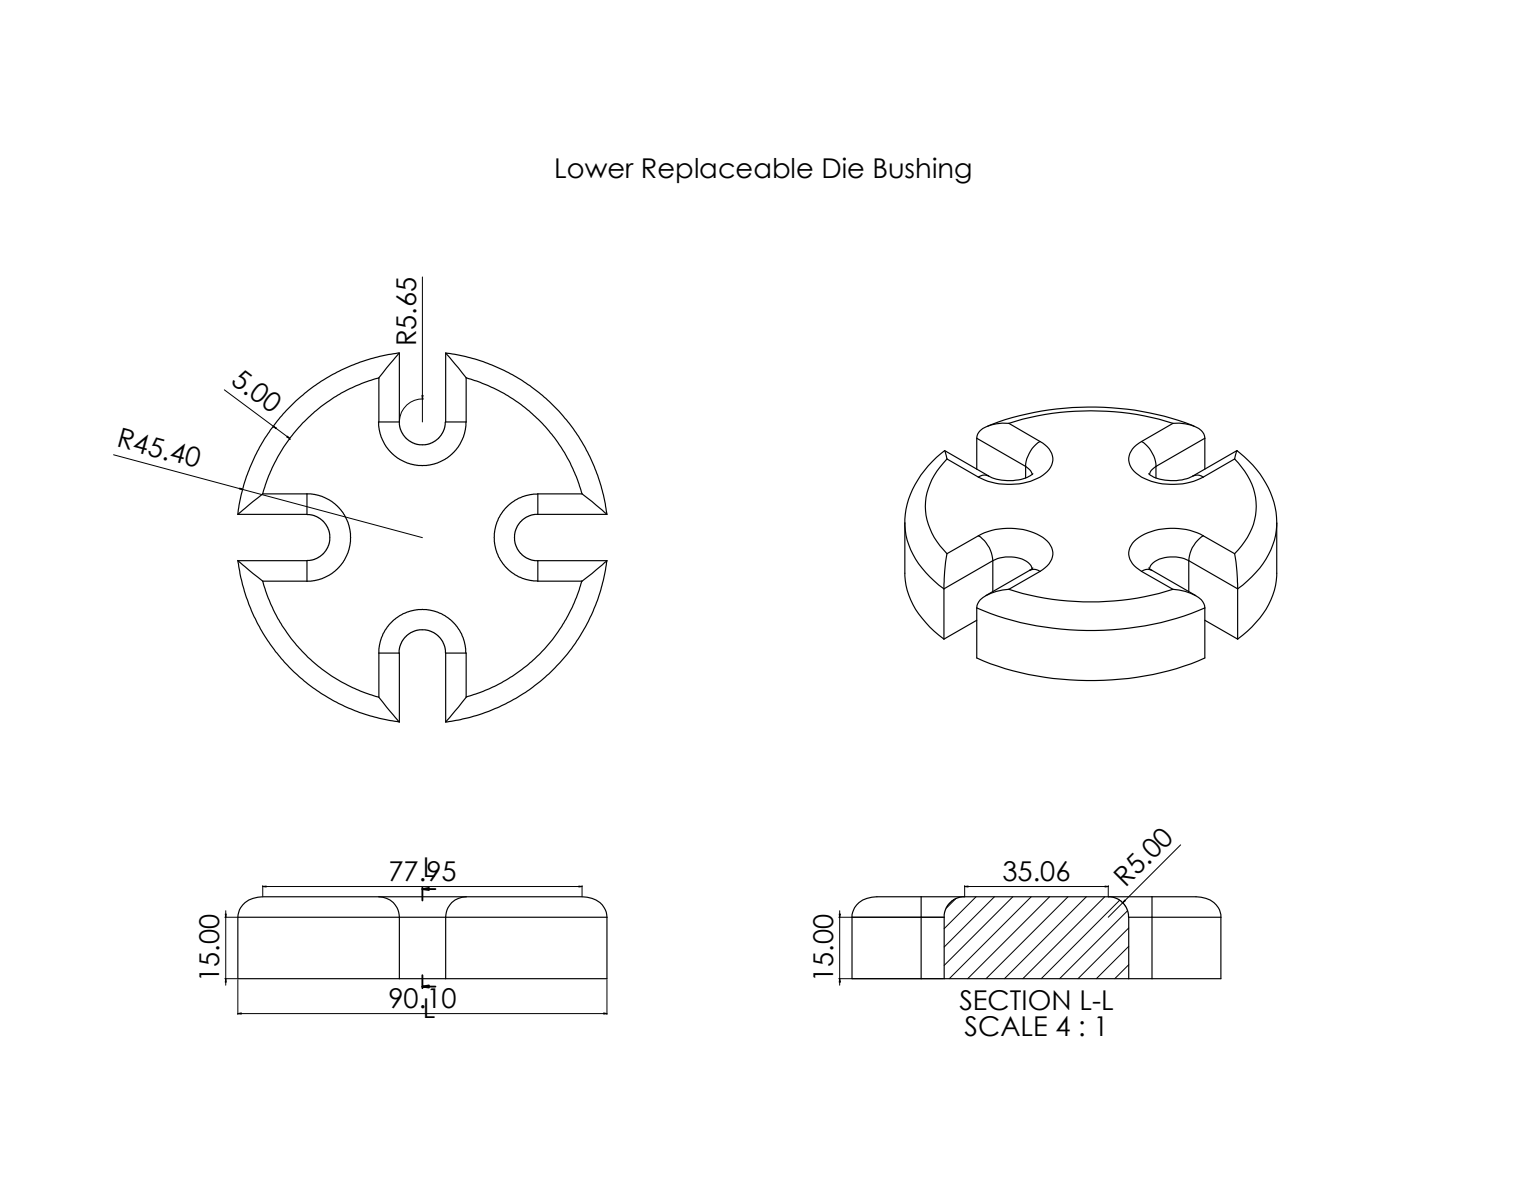
ISO-10303-21;
HEADER;
FILE_DESCRIPTION (('STEP AP214'),
    '1' );
FILE_NAME ('Lower Replaceable Die Bushing.step',
    '2026-10-21T18:33:49',
    ( '' ),
    ( '' ),
    'SwSTEP 2.0',
    'SolidWorks 2025',
    '' );
FILE_SCHEMA (( 'AUTOMOTIVE_DESIGN' ));
ENDSEC;

DATA;
#18=CARTESIAN_POINT ( 'NONE',  ( -78.51801170372752381, -91.96846159163192169, 42.55230335834794175 ) ) ;
#24=CARTESIAN_POINT ( 'NONE',  ( -110.0337185876616815, -91.08930958056578220, -10.39386245929468444 ) ) ;
#38=CARTESIAN_POINT ( 'NONE',  ( -27.30335599338096841, -92.58099833983887095, 7.070576347711331699 ) ) ;
#39=DIRECTION ( 'NONE',  ( 3.469446951953611033E-15, 0.000000000000000000, -1.000000000000000000 ) ) ;
#48=DIRECTION ( 'NONE',  ( -1.000000000000000000, 0.000000000000000000, 0.000000000000000000 ) ) ;
#60=VERTEX_POINT ( 'NONE', #5921 ) ;
#117=DIRECTION ( 'NONE',  ( 0.000000000000000000, 1.000000000000000000, -0.000000000000000000 ) ) ;
#121=CARTESIAN_POINT ( 'NONE',  ( -115.7702289486887537, -95.65021661331556402, -5.654315315326000402 ) ) ;
#129=FACE_OUTER_BOUND ( 'NONE', #15736, .T. ) ;
#153=ORIENTED_EDGE ( 'NONE', *, *, #7643, .F. ) ;
#166=PLANE ( 'NONE',  #9698 ) ;
#184=CARTESIAN_POINT ( 'NONE',  ( -64.80066835027049876, -94.42547236494613117, -44.74948972093426391 ) ) ;
#208=CARTESIAN_POINT ( 'NONE',  ( -80.32997185471272417, -91.18731257919070288, 40.31990080433438095 ) ) ;
#212=CARTESIAN_POINT ( 'NONE',  ( -114.8884567811962967, -93.39009998357855125, -6.425136209964025902 ) ) ;
#215=ADVANCED_FACE ( 'NONE', ( #695 ), #10288, .T. ) ;
#221=CARTESIAN_POINT ( 'NONE',  ( -81.37409655828265898, -96.08423613455721579, -2.623087607583323579E-13 ) ) ;
#233=EDGE_CURVE ( 'NONE', #4074, #17713, #2000, .T. ) ;
#247=EDGE_LOOP ( 'NONE', ( #1699, #2209, #13687, #4336 ) ) ;
#251=AXIS2_PLACEMENT_3D ( 'NONE', #13885, #4066, #1079 ) ;
#273=ORIENTED_EDGE ( 'NONE', *, *, #7918, .F. ) ;
#275=ORIENTED_EDGE ( 'NONE', *, *, #8832, .T. ) ;
#285=CARTESIAN_POINT ( 'NONE',  ( -80.85270481229034090, -91.10977358899566525, 39.65137850708985923 ) ) ;
#290=DIRECTION ( 'NONE',  ( 0.000000000000000000, 1.000000000000000000, -0.000000000000000000 ) ) ;
#336=CARTESIAN_POINT ( 'NONE',  ( 0.000000000000000000, -111.0842361345572158, 0.000000000000000000 ) ) ;
#343=DIRECTION ( 'NONE',  ( -0.000000000000000000, -1.000000000000000000, 0.000000000000000000 ) ) ;
#373=ADVANCED_FACE ( 'NONE', ( #129 ), #745, .T. ) ;
#380=CARTESIAN_POINT ( 'NONE',  ( -81.37409655828265898, -96.08423613455721579, -8.525034724645805924E-13 ) ) ;
#398=LINE ( 'NONE', #4246, #4265 ) ;
#400=CARTESIAN_POINT ( 'NONE',  ( -28.16748190072492974, -91.96845925178433845, 7.798233810088259332 ) ) ;
#432=VECTOR ( 'NONE', #18327, 1000.000000000000000 ) ;
#460=DIRECTION ( 'NONE',  ( -0.000000000000000000, -1.000000000000000000, -0.000000000000000000 ) ) ;
#467=ORIENTED_EDGE ( 'NONE', *, *, #4024, .T. ) ;
#480=CARTESIAN_POINT ( 'NONE',  ( -76.37409655828265898, -111.0842361345572158, -2.461913000519969422E-13 ) ) ;
#513=VERTEX_POINT ( 'NONE', #15067 ) ;
#516=ORIENTED_EDGE ( 'NONE', *, *, #6768, .F. ) ;
#582=DIRECTION ( 'NONE',  ( -1.000000000000000000, 0.000000000000000000, -6.950654929607132427E-15 ) ) ;
#614=ORIENTED_EDGE ( 'NONE', *, *, #15108, .F. ) ;
#620=CYLINDRICAL_SURFACE ( 'NONE', #5187, 5.654315315325682434 ) ;
#640=CARTESIAN_POINT ( 'NONE',  ( -42.53669312409158465, -96.08423613455721579, 5.204170427930421283E-15 ) ) ;
#642=EDGE_CURVE ( 'NONE', #11067, #11836, #18161, .T. ) ;
#660=CARTESIAN_POINT ( 'NONE',  ( -98.90286936182226896, -91.08423613455721579, -10.65431531532588316 ) ) ;
#662=CARTESIAN_POINT ( 'NONE',  ( -76.37409655828280108, -111.0842361345572158, 45.05044770573179846 ) ) ;
#690=ADVANCED_FACE ( 'NONE', ( #9649 ), #1237, .F. ) ;
#695=FACE_OUTER_BOUND ( 'NONE', #12047, .T. ) ;
#696=CARTESIAN_POINT ( 'NONE',  ( -42.53669312409158465, -96.08423613455721579, 5.204170427930421283E-15 ) ) ;
#701=DIRECTION ( 'NONE',  ( -0.000000000000000000, -1.000000000000000000, -0.000000000000000000 ) ) ;
#705=DIRECTION ( 'NONE',  ( 0.000000000000000000, 0.000000000000000000, 1.000000000000000000 ) ) ;
#745=TOROIDAL_SURFACE ( 'NONE', #11214, 40.40389983439752086, 5.000000000000000000 ) ;
#749=VECTOR ( 'NONE', #11083, 1000.000000000000000 ) ;
#759=DIRECTION ( 'NONE',  ( 9.117856171852156377E-15, 0.000000000000000000, 1.000000000000000000 ) ) ;
#763=CARTESIAN_POINT ( 'NONE',  ( -31.57667891805219895, -91.08423613455724421, -10.52509945732311891 ) ) ;
#787=EDGE_LOOP ( 'NONE', ( #8636, #4060, #891, #3393 ) ) ;
#799=DIRECTION ( 'NONE',  ( 1.000000000000000000, 0.000000000000000000, -0.000000000000000000 ) ) ;
#800=VERTEX_POINT ( 'NONE', #13028 ) ;
#830=ORIENTED_EDGE ( 'NONE', *, *, #10988, .T. ) ;
#836=LINE ( 'NONE', #4020, #9670 ) ;
#853=DIRECTION ( 'NONE',  ( 0.000000000000000000, 1.000000000000000000, -0.000000000000000000 ) ) ;
#867=B_SPLINE_CURVE_WITH_KNOTS ( 'NONE', 3,
 ( #14957, #763, #6351, #1047, #10957, #8142, #9362, #2435, #16641, #15059, #7957, #5140, #10857, #13758, #16454, #9455, #18156, #6644, #12083, #12462 ),
 .UNSPECIFIED., .F., .F.,
 ( 4, 2, 2, 2, 2, 2, 2, 2, 2, 4 ),
 ( -1.439925654488394098E-05, 0.0006244272253376518481, 0.001263253707220187783, 0.002540906670985255533, 0.003818559634750323065, 0.005096212598515390164, 0.006373865562280457697, 0.007651518526045524363, 0.008929171489810592763, 0.01020682445357565943 ),
 .UNSPECIFIED. ) ;
#875=CARTESIAN_POINT ( 'NONE',  ( -70.71978124295696944, -96.08423613455721579, 5.204170427930421283E-15 ) ) ;
#888=CARTESIAN_POINT ( 'NONE',  ( -81.11364370225096820, -91.08930958056581062, -39.31393734470488255 ) ) ;
#891=ORIENTED_EDGE ( 'NONE', *, *, #12147, .T. ) ;
#911=VECTOR ( 'NONE', #6055, 1000.000000000000000 ) ;
#939=EDGE_CURVE ( 'NONE', #10198, #60, #13560, .T. ) ;
#966=CARTESIAN_POINT ( 'NONE',  ( -115.7702289486888247, -96.08423613455721579, 5.654315315325360913 ) ) ;
#976=CYLINDRICAL_SURFACE ( 'NONE', #17426, 45.40389983439752086 ) ;
#1015=CARTESIAN_POINT ( 'NONE',  ( -60.06546592763143622, -91.08423613455721579, 38.97384619189705290 ) ) ;
#1016=CARTESIAN_POINT ( 'NONE',  ( -63.40980125876075135, -92.35432432510552303, 43.13417342538335930 ) ) ;
#1043=DIRECTION ( 'NONE',  ( 0.000000000000000000, 1.000000000000000000, -0.000000000000000000 ) ) ;
#1047=CARTESIAN_POINT ( 'NONE',  ( -31.06841040534018106, -91.10977296152353233, -10.13292952605206310 ) ) ;
#1055=ADVANCED_FACE ( 'NONE', ( #3537 ), #14940, .T. ) ;
#1058=UNCERTAINTY_MEASURE_WITH_UNIT (LENGTH_MEASURE( 1.000000000000000082E-05 ), #12203, 'distance_accuracy_value', 'NONE');
#1079=DIRECTION ( 'NONE',  ( 0.000000000000000000, 0.000000000000000000, -1.000000000000000000 ) ) ;
#1087=CARTESIAN_POINT ( 'NONE',  ( -70.71978124295668522, -96.08423613455721579, -17.52877280353970235 ) ) ;
#1089=CARTESIAN_POINT ( 'NONE',  ( -30.06971094502080177, -91.24992749556385263, 9.348345296714491326 ) ) ;
#1115=VERTEX_POINT ( 'NONE', #16826 ) ;
#1116=CARTESIAN_POINT ( 'NONE',  ( -62.67046908522836191, -91.80659809767264790, 42.25010775664332385 ) ) ;
#1128=DIRECTION ( 'NONE',  ( -0.000000000000000000, -1.000000000000000000, -0.000000000000000000 ) ) ;
#1157=CARTESIAN_POINT ( 'NONE',  ( -70.71978124295696944, -96.08423613455721579, 5.204170427930421283E-15 ) ) ;
#1166=DIRECTION ( 'NONE',  ( 0.000000000000000000, 0.000000000000000000, 1.000000000000000000 ) ) ;
#1214=DIRECTION ( 'NONE',  ( 0.000000000000000000, -0.000000000000000000, 1.000000000000000000 ) ) ;
#1237=CYLINDRICAL_SURFACE ( 'NONE', #13579, 5.654315315325682434 ) ;
#1244=ORIENTED_EDGE ( 'NONE', *, *, #8704, .T. ) ;
#1273=LINE ( 'NONE', #6877, #3065 ) ;
#1297=DIRECTION ( 'NONE',  ( 0.000000000000000000, 0.000000000000000000, 1.000000000000000000 ) ) ;
#1307=EDGE_CURVE ( 'NONE', #800, #4074, #8827, .T. ) ;
#1325=LINE ( 'NONE', #9738, #8125 ) ;
#1351=ORIENTED_EDGE ( 'NONE', *, *, #2145, .T. ) ;
#1352=AXIS2_PLACEMENT_3D ( 'NONE', #4171, #12879, #17171 ) ;
#1385=DIRECTION ( 'NONE',  ( -0.000000000000000000, -1.000000000000000000, -0.000000000000000000 ) ) ;
#1398=LINE ( 'NONE', #18508, #12882 ) ;
#1404=ORIENTED_EDGE ( 'NONE', *, *, #16960, .T. ) ;
#1408=CARTESIAN_POINT ( 'NONE',  ( -62.15805688404110185, -91.53392936304808813, -41.62626455281442617 ) ) ;
#1453=LINE ( 'NONE', #7252, #16398 ) ;
#1518=CARTESIAN_POINT ( 'NONE',  ( -98.90286936182226896, -96.08423613455721579, -10.65431531532588494 ) ) ;
#1520=CARTESIAN_POINT ( 'NONE',  ( -80.06812138002696599, -91.24992890033500714, 40.65007677557128574 ) ) ;
#1528=ADVANCED_FACE ( 'NONE', ( #17112 ), #14234, .T. ) ;
#1541=AXIS2_PLACEMENT_3D ( 'NONE', #17995, #9123, #14899 ) ;
#1567=DIRECTION ( 'NONE',  ( 0.000000000000000000, 0.000000000000000000, 1.000000000000000000 ) ) ;
#1571=CARTESIAN_POINT ( 'NONE',  ( -65.06546592763082515, -91.08423613455721579, -45.05044770573174873 ) ) ;
#1577=ORIENTED_EDGE ( 'NONE', *, *, #16595, .T. ) ;
#1615=CARTESIAN_POINT ( 'NONE',  ( -111.0396820472913220, -91.18731257919070288, -9.610190611755886181 ) ) ;
#1629=EDGE_LOOP ( 'NONE', ( #8679, #16373, #14384, #17205 ) ) ;
#1647=CARTESIAN_POINT ( 'NONE',  ( -76.37409655828275845, -96.08423613455721579, 28.18308811886536347 ) ) ;
#1699=ORIENTED_EDGE ( 'NONE', *, *, #16467, .T. ) ;
#1712=DIRECTION ( 'NONE',  ( 0.000000000000000000, 0.000000000000000000, 1.000000000000000000 ) ) ;
#1713=FACE_OUTER_BOUND ( 'NONE', #7475, .T. ) ;
#1732=DIRECTION ( 'NONE',  ( -1.000000000000000000, 0.000000000000000000, -3.223492141267075737E-15 ) ) ;
#1740=PLANE ( 'NONE',  #13721 ) ;
#1746=DIRECTION ( 'NONE',  ( -0.000000000000000000, -1.000000000000000000, -0.000000000000000000 ) ) ;
#1774=CYLINDRICAL_SURFACE ( 'NONE', #16267, 4.999999999999997335 ) ;
#1778=ADVANCED_FACE ( 'NONE', ( #3809 ), #13608, .T. ) ;
#1780=CARTESIAN_POINT ( 'NONE',  ( -79.54423376290981196, -91.42293805878658475, 41.30286037549874578 ) ) ;
#1781=VECTOR ( 'NONE', #15202, 1000.000000000000000 ) ;
#1822=ORIENTED_EDGE ( 'NONE', *, *, #10528, .T. ) ;
#1840=DIRECTION ( 'NONE',  ( 0.000000000000000000, 0.000000000000000000, 1.000000000000000000 ) ) ;
#1855=ADVANCED_FACE ( 'NONE', ( #17513 ), #8919, .T. ) ;
#1891=DIRECTION ( 'NONE',  ( 0.000000000000000000, 0.000000000000000000, 1.000000000000000000 ) ) ;
#1942=EDGE_CURVE ( 'NONE', #14058, #17058, #10586, .T. ) ;
#1992=CARTESIAN_POINT ( 'NONE',  ( -114.1362093120869758, -92.58100082067042536, 7.070573948080970617 ) ) ;
#2000=LINE ( 'NONE', #10791, #16263 ) ;
#2006=FACE_OUTER_BOUND ( 'NONE', #3138, .T. ) ;
#2009=CARTESIAN_POINT ( 'NONE',  ( -0.000000000000000000, -111.0842361345572158, -5.654315315325675328 ) ) ;
#2013=CARTESIAN_POINT ( 'NONE',  ( -80.32997185471215573, -91.18731257919071709, -40.31990080433450885 ) ) ;
#2061=DIRECTION ( 'NONE',  ( 0.000000000000000000, 1.000000000000000000, -0.000000000000000000 ) ) ;
#2075=PLANE ( 'NONE',  #3272 ) ;
#2100=CARTESIAN_POINT ( 'NONE',  ( -60.06546592763139358, -96.08423613455721579, 28.18308811886542742 ) ) ;
#2132=FACE_OUTER_BOUND ( 'NONE', #14459, .T. ) ;
#2145=EDGE_CURVE ( 'NONE', #11655, #5840, #14937, .T. ) ;
#2161=DIRECTION ( 'NONE',  ( -0.000000000000000000, -1.000000000000000000, 0.000000000000000000 ) ) ;
#2185=CARTESIAN_POINT ( 'NONE',  ( -70.71978124295668522, -96.08423613455721579, -28.18308811886538479 ) ) ;
#2202=CARTESIAN_POINT ( 'NONE',  ( -76.42964172313168092, -95.23217669033338950, -44.98760873426162021 ) ) ;
#2209=ORIENTED_EDGE ( 'NONE', *, *, #15596, .F. ) ;
#2235=ORIENTED_EDGE ( 'NONE', *, *, #9721, .T. ) ;
#2276=DIRECTION ( 'NONE',  ( 0.000000000000000000, 0.000000000000000000, -1.000000000000000000 ) ) ;
#2280=CYLINDRICAL_SURFACE ( 'NONE', #15870, 5.000000000000000000 ) ;
#2289=CARTESIAN_POINT ( 'NONE',  ( -78.76908973550854398, -91.80660034481559251, -42.25011218277860081 ) ) ;
#2334=TOROIDAL_SURFACE ( 'NONE', #17864, 40.40389983439752086, 5.000000000000000000 ) ;
#2364=FACE_OUTER_BOUND ( 'NONE', #17216, .T. ) ;
#2370=ORIENTED_EDGE ( 'NONE', *, *, #7643, .T. ) ;
#2373=DIRECTION ( 'NONE',  ( -0.000000000000000000, -1.000000000000000000, -0.000000000000000000 ) ) ;
#2379=DIRECTION ( 'NONE',  ( 0.000000000000000000, 1.000000000000000000, -0.000000000000000000 ) ) ;
#2403=EDGE_CURVE ( 'NONE', #5840, #5095, #13540, .T. ) ;
#2405=CARTESIAN_POINT ( 'NONE',  ( -62.15805688404169160, -91.53392936304808813, 41.62626455281458249 ) ) ;
#2430=EDGE_CURVE ( 'NONE', #16406, #17849, #17359, .T. ) ;
#2435=CARTESIAN_POINT ( 'NONE',  ( -29.41692657362415275, -91.42293623445492301, -8.824457138344822482 ) ) ;
#2458=DIRECTION ( 'NONE',  ( 0.000000000000000000, 0.000000000000000000, 1.000000000000000000 ) ) ;
#2460=CYLINDRICAL_SURFACE ( 'NONE', #251, 5.000000000000000000 ) ;
#2471=CARTESIAN_POINT ( 'NONE',  ( -30.39988730823796104, -91.18731141006421126, 9.610196039195450624 ) ) ;
#2490=DIRECTION ( 'NONE',  ( 0.000000000000000000, 1.000000000000000000, -0.000000000000000000 ) ) ;
#2502=CARTESIAN_POINT ( 'NONE',  ( -98.90286936182243949, -91.08423613455721579, 10.65431531532547638 ) ) ;
#2527=VECTOR ( 'NONE', #14900, 1000.000000000000000 ) ;
#2531=LINE ( 'NONE', #12545, #15899 ) ;
#2554=CYLINDRICAL_SURFACE ( 'NONE', #6659, 5.654315315325680658 ) ;
#2559=ORIENTED_EDGE ( 'NONE', *, *, #6394, .T. ) ;
#2592=EDGE_LOOP ( 'NONE', ( #2918, #8135, #9443, #11259 ) ) ;
#2606=CARTESIAN_POINT ( 'NONE',  ( -42.53669312409158465, -111.0842361345572158, -5.654315315325675328 ) ) ;
#2666=LINE ( 'NONE', #15391, #749 ) ;
#2691=DIRECTION ( 'NONE',  ( -1.000000000000000000, 0.000000000000000000, -4.029365176583844474E-15 ) ) ;
#2712=AXIS2_PLACEMENT_3D ( 'NONE', #640, #4570, #3346 ) ;
#2738=( GEOMETRIC_REPRESENTATION_CONTEXT ( 3 ) GLOBAL_UNCERTAINTY_ASSIGNED_CONTEXT ( ( #1058 ) ) GLOBAL_UNIT_ASSIGNED_CONTEXT ( ( #12203, #9578, #17895 ) ) REPRESENTATION_CONTEXT ( 'NONE', 'WORKASPACE' ) );
#2744=CARTESIAN_POINT ( 'NONE',  ( -115.7073899772185257, -95.23217669033341792, -5.709860480175484199 ) ) ;
#2763=CARTESIAN_POINT ( 'NONE',  ( -70.71978124295668522, -96.08423613455721579, -22.52877280353970235 ) ) ;
#2772=ORIENTED_EDGE ( 'NONE', *, *, #939, .F. ) ;
#2780=ORIENTED_EDGE ( 'NONE', *, *, #9396, .T. ) ;
#2813=VECTOR ( 'NONE', #16740, 1000.000000000000000 ) ;
#2820=CIRCLE ( 'NONE', #6674, 5.654315315325680658 ) ;
#2840=CARTESIAN_POINT ( 'NONE',  ( 3.930119462001817841E-14, -111.0842361345572158, -5.654315315325195712 ) ) ;
#2852=CARTESIAN_POINT ( 'NONE',  ( -76.37409655828280108, -91.08423613455721579, 45.05044770573179846 ) ) ;
#2882=ADVANCED_FACE ( 'NONE', ( #18185 ), #976, .T. ) ;
#2904=CARTESIAN_POINT ( 'NONE',  ( -60.32591256472567665, -91.08930925317537231, -39.31392926885246197 ) ) ;
#2910=ORIENTED_EDGE ( 'NONE', *, *, #14027, .F. ) ;
#2918=ORIENTED_EDGE ( 'NONE', *, *, #8704, .F. ) ;
#2924=VERTEX_POINT ( 'NONE', #14169 ) ;
#2930=CARTESIAN_POINT ( 'NONE',  ( -115.3009539377894015, -94.06000857856476216, -6.066633078422342784 ) ) ;
#2931=ORIENTED_EDGE ( 'NONE', *, *, #4659, .F. ) ;
#2939=CARTESIAN_POINT ( 'NONE',  ( -25.73217265163131984, -95.23217577251028843, 5.709860606646938841 ) ) ;
#2949=ORIENTED_EDGE ( 'NONE', *, *, #11587, .T. ) ;
#2958=CARTESIAN_POINT ( 'NONE',  ( -115.7702289486887395, -111.0842361345572158, -5.654315315326000402 ) ) ;
#2984=EDGE_CURVE ( 'NONE', #9931, #14963, #7408, .T. ) ;
#3012=VECTOR ( 'NONE', #460, 1000.000000000000000 ) ;
#3018=ORIENTED_EDGE ( 'NONE', *, *, #14027, .T. ) ;
#3019=CARTESIAN_POINT ( 'NONE',  ( -111.3698580185282054, -91.24992890033504978, -9.348340137070142219 ) ) ;
#3023=ORIENTED_EDGE ( 'NONE', *, *, #9031, .T. ) ;
#3033=CARTESIAN_POINT ( 'NONE',  ( -76.37409655828219002, -111.0842361345572158, -45.05044770573186952 ) ) ;
#3034=CIRCLE ( 'NONE', #18273, 5.654315315325682434 ) ;
#3049=DIRECTION ( 'NONE',  ( -1.000000000000000000, 0.000000000000000000, 0.000000000000000000 ) ) ;
#3065=VECTOR ( 'NONE', #18297, 1000.000000000000000 ) ;
#3124=CARTESIAN_POINT ( 'NONE',  ( -25.66933353722515676, -96.08423613455721579, 5.654315315325685987 ) ) ;
#3138=EDGE_LOOP ( 'NONE', ( #7995, #4313, #2910, #273 ) ) ;
#3140=ORIENTED_EDGE ( 'NONE', *, *, #5509, .T. ) ;
#3144=CARTESIAN_POINT ( 'NONE',  ( -42.53669312409158465, -91.08423613455721579, -10.65431531532567533 ) ) ;
#3159=FACE_OUTER_BOUND ( 'NONE', #17830, .T. ) ;
#3164=EDGE_CURVE ( 'NONE', #60, #3192, #9096, .T. ) ;
#3190=CARTESIAN_POINT ( 'NONE',  ( -70.71978124295696944, -111.0842361345572158, 5.204170427930421283E-15 ) ) ;
#3192=VERTEX_POINT ( 'NONE', #3656 ) ;
#3267=DIRECTION ( 'NONE',  ( -0.000000000000000000, -1.000000000000000000, -0.000000000000000000 ) ) ;
#3272=AXIS2_PLACEMENT_3D ( 'NONE', #6462, #3661, #9373 ) ;
#3278=AXIS2_PLACEMENT_3D ( 'NONE', #15467, #10976, #2458 ) ;
#3305=AXIS2_PLACEMENT_3D ( 'NONE', #2100, #7809, #9127 ) ;
#3311=PLANE ( 'NONE',  #5987 ) ;
#3341=CARTESIAN_POINT ( 'NONE',  ( -42.53669312409158465, -96.08423613455721579, -5.654315315325675328 ) ) ;
#3346=DIRECTION ( 'NONE',  ( 0.000000000000000000, 0.000000000000000000, 1.000000000000000000 ) ) ;
#3380=ORIENTED_EDGE ( 'NONE', *, *, #2984, .F. ) ;
#3384=CARTESIAN_POINT ( 'NONE',  ( -115.3009539377894868, -94.06000857856477637, 6.066633078421709513 ) ) ;
#3392=EDGE_LOOP ( 'NONE', ( #14489, #5848, #17476, #6477 ) ) ;
#3393=ORIENTED_EDGE ( 'NONE', *, *, #17820, .T. ) ;
#3413=CARTESIAN_POINT ( 'NONE',  ( -78.02975850117498169, -92.35432678654406402, -43.13417664947088070 ) ) ;
#3420=EDGE_CURVE ( 'NONE', #13598, #16250, #9844, .T. ) ;
#3453=APPLICATION_CONTEXT ( 'automotive_design' ) ;
#3485=CARTESIAN_POINT ( 'NONE',  ( -112.9698934257355631, -91.80660034481556409, 8.049308492551670469 ) ) ;
#3499=ORIENTED_EDGE ( 'NONE', *, *, #9626, .F. ) ;
#3524=CARTESIAN_POINT ( 'NONE',  ( -65.06546592763150727, -95.65021616327639720, 45.05044770573186952 ) ) ;
#3535=ORIENTED_EDGE ( 'NONE', *, *, #4255, .F. ) ;
#3537=FACE_OUTER_BOUND ( 'NONE', #6250, .T. ) ;
#3570=CARTESIAN_POINT ( 'NONE',  ( -113.8539578924278288, -92.35432678654406402, 7.309977258218128604 ) ) ;
#3593=CARTESIAN_POINT ( 'NONE',  ( 0.000000000000000000, -111.0842361345572158, 5.654315315325685987 ) ) ;
#3602=B_SPLINE_CURVE_WITH_KNOTS ( 'NONE', 3,
 ( #18392, #15282, #5277, #10989, #11080, #2471, #1089, #12497, #18191, #4511, #400, #6088, #38, #7245, #11464, #10053, #12966, #2939, #4421, #3124 ),
 .UNSPECIFIED., .F., .F.,
 ( 4, 2, 2, 2, 2, 2, 2, 2, 2, 4 ),
 ( -1.439925654488394098E-05, 0.0006244272253376518481, 0.001263253707220187783, 0.002540906670985255533, 0.003818559634750323065, 0.005096212598515390164, 0.006373865562280457697, 0.007651518526045524363, 0.008929171489810592763, 0.01020682445357565943 ),
 .UNSPECIFIED. ) ;
#3607=ORIENTED_EDGE ( 'NONE', *, *, #11354, .F. ) ;
#3608=EDGE_CURVE ( 'NONE', #11153, #4979, #11030, .T. ) ;
#3616=CIRCLE ( 'NONE', #1541, 4.999999999999997335 ) ;
#3656=CARTESIAN_POINT ( 'NONE',  ( -65.06546592763099568, -111.0842361345572158, -28.18308811886532084 ) ) ;
#3661=DIRECTION ( 'NONE',  ( 6.950654929607132427E-15, 0.000000000000000000, -1.000000000000000000 ) ) ;
#3663=DIRECTION ( 'NONE',  ( -0.000000000000000000, -1.000000000000000000, -0.000000000000000000 ) ) ;
#3681=AXIS2_PLACEMENT_3D ( 'NONE', #16726, #1043, #8035 ) ;
#3692=CARTESIAN_POINT ( 'NONE',  ( -65.06546592763082515, -96.08423613455721579, -45.05044770573174873 ) ) ;
#3705=CARTESIAN_POINT ( 'NONE',  ( -79.28150129717847960, -91.53393135689863414, -41.62626982970579803 ) ) ;
#3710=VERTEX_POINT ( 'NONE', #9029 ) ;
#3725=AXIS2_PLACEMENT_3D ( 'NONE', #5512, #16718, #9731 ) ;
#3745=CARTESIAN_POINT ( 'NONE',  ( -65.06546592763139358, -91.08423613455721579, 28.18308811886540610 ) ) ;
#3775=CARTESIAN_POINT ( 'NONE',  ( -70.71978124295696944, -91.08423613455721579, 5.204170427930421283E-15 ) ) ;
#3787=ORIENTED_EDGE ( 'NONE', *, *, #15596, .T. ) ;
#3809=FACE_OUTER_BOUND ( 'NONE', #2592, .T. ) ;
#3816=VERTEX_POINT ( 'NONE', #2958 ) ;
#3824=VECTOR ( 'NONE', #17984, 1000.000000000000000 ) ;
#3825=DIRECTION ( 'NONE',  ( -0.000000000000000000, -1.000000000000000000, -0.000000000000000000 ) ) ;
#3830=ORIENTED_EDGE ( 'NONE', *, *, #9959, .T. ) ;
#3833=ORIENTED_EDGE ( 'NONE', *, *, #13387, .T. ) ;
#3855=DIRECTION ( 'NONE',  ( 0.000000000000000000, 0.000000000000000000, 1.000000000000000000 ) ) ;
#3905=CARTESIAN_POINT ( 'NONE',  ( -61.37143594624264153, -91.24992749556382421, 40.65007029793621030 ) ) ;
#3912=CIRCLE ( 'NONE', #8948, 40.40389983439752086 ) ;
#3954=DIRECTION ( 'NONE',  ( 0.000000000000000000, 1.000000000000000000, -0.000000000000000000 ) ) ;
#3989=CARTESIAN_POINT ( 'NONE',  ( -42.53669312409158465, -111.0842361345572158, 5.654315315325685987 ) ) ;
#4020=CARTESIAN_POINT ( 'NONE',  ( -98.90286936182239685, -91.08423613455721579, 5.654315315325477265 ) ) ;
#4024=EDGE_CURVE ( 'NONE', #7404, #16572, #17020, .T. ) ;
#4027=EDGE_CURVE ( 'NONE', #14163, #4979, #1453, .T. ) ;
#4041=CARTESIAN_POINT ( 'NONE',  ( -109.6936274348540508, -91.08423613455721579, 10.65431531532540177 ) ) ;
#4042=ORIENTED_EDGE ( 'NONE', *, *, #9626, .T. ) ;
#4060=ORIENTED_EDGE ( 'NONE', *, *, #7425, .T. ) ;
#4066=DIRECTION ( 'NONE',  ( 1.000000000000000000, 0.000000000000000000, 0.000000000000000000 ) ) ;
#4074=VERTEX_POINT ( 'NONE', #15845 ) ;
#4114=CARTESIAN_POINT ( 'NONE',  ( -65.00992063630958739, -95.23217577251027421, -44.98760859132558210 ) ) ;
#4126=LINE ( 'NONE', #9929, #6576 ) ;
#4171=CARTESIAN_POINT ( 'NONE',  ( -81.37409655828237476, -96.08423613455721579, -28.18308811886549847 ) ) ;
#4183=DIRECTION ( 'NONE',  ( -0.000000000000000000, -1.000000000000000000, 0.000000000000000000 ) ) ;
#4223=VECTOR ( 'NONE', #18195, 1000.000000000000000 ) ;
#4237=CARTESIAN_POINT ( 'NONE',  ( -115.4692715616776866, -94.42547395655694231, -5.919112368231730592 ) ) ;
#4246=CARTESIAN_POINT ( 'NONE',  ( 0.000000000000000000, -91.08423613455721579, -10.65431531532567710 ) ) ;
#4255=EDGE_CURVE ( 'NONE', #15074, #7696, #10153, .T. ) ;
#4265=VECTOR ( 'NONE', #17151, 1000.000000000000000 ) ;
#4282=CARTESIAN_POINT ( 'NONE',  ( -60.06546592763139358, -91.08423613455721579, 28.18308811886542742 ) ) ;
#4286=CARTESIAN_POINT ( 'NONE',  ( -70.71978124295696944, -96.08423613455721579, 5.204170427930421283E-15 ) ) ;
#4304=EDGE_LOOP ( 'NONE', ( #3023, #8778, #14360, #14095 ) ) ;
#4313=ORIENTED_EDGE ( 'NONE', *, *, #4027, .F. ) ;
#4336=ORIENTED_EDGE ( 'NONE', *, *, #8337, .F. ) ;
#4347=DIRECTION ( 'NONE',  ( 0.000000000000000000, 0.000000000000000000, 1.000000000000000000 ) ) ;
#4350=EDGE_CURVE ( 'NONE', #6267, #17849, #16714, .T. ) ;
#4421=CARTESIAN_POINT ( 'NONE',  ( -25.66933353722516031, -95.65021616327642562, 5.654315315325686875 ) ) ;
#4499=TOROIDAL_SURFACE ( 'NONE', #2712, 10.65431531532567888, 5.000000000000000000 ) ;
#4509=DIRECTION ( 'NONE',  ( -0.000000000000000000, -1.000000000000000000, -0.000000000000000000 ) ) ;
#4511=CARTESIAN_POINT ( 'NONE',  ( -28.46967348631369177, -91.80659809767261947, 8.049312157728774508 ) ) ;
#4530=CARTESIAN_POINT ( 'NONE',  ( -70.71978124295668522, -91.08423613455721579, -28.18308811886538479 ) ) ;
#4532=ORIENTED_EDGE ( 'NONE', *, *, #4255, .T. ) ;
#4570=DIRECTION ( 'NONE',  ( 0.000000000000000000, 1.000000000000000000, -0.000000000000000000 ) ) ;
#4572=VECTOR ( 'NONE', #1746, 1000.000000000000000 ) ;
#4590=CARTESIAN_POINT ( 'NONE',  ( -81.24478565583312673, -91.08423613455723000, 39.14322682088972272 ) ) ;
#4618=ORIENTED_EDGE ( 'NONE', *, *, #8832, .F. ) ;
#4638=AXIS2_PLACEMENT_3D ( 'NONE', #7114, #12821, #11420 ) ;
#4659=EDGE_CURVE ( 'NONE', #13953, #12828, #17629, .T. ) ;
#4679=DIRECTION ( 'NONE',  ( 0.000000000000000000, 1.000000000000000000, -0.000000000000000000 ) ) ;
#4684=EDGE_CURVE ( 'NONE', #513, #12828, #5077, .T. ) ;
#4686=CARTESIAN_POINT ( 'NONE',  ( -70.71978124295668522, -91.08423613455721579, -28.18308811886538479 ) ) ;
#4709=FACE_OUTER_BOUND ( 'NONE', #9933, .T. ) ;
#4711=FACE_OUTER_BOUND ( 'NONE', #13237, .T. ) ;
#4718=VERTEX_POINT ( 'NONE', #12170 ) ;
#4724=SHAPE_REPRESENTATION_RELATIONSHIP ( 'NONE' , 'NONE' ,  #13055, #7691 ) ;
#4735=FACE_OUTER_BOUND ( 'NONE', #8532, .T. ) ;
#4759=DIRECTION ( 'NONE',  ( 0.000000000000000000, 0.000000000000000000, 1.000000000000000000 ) ) ;
#4774=CARTESIAN_POINT ( 'NONE',  ( -70.71978124295696944, -91.08423613455721579, 5.204170427930421283E-15 ) ) ;
#4775=DIRECTION ( 'NONE',  ( 1.047634945911799279E-14, 0.000000000000000000, -1.000000000000000000 ) ) ;
#4810=CARTESIAN_POINT ( 'NONE',  ( -76.37409655828220423, -95.65021661331557823, -45.05044770573186952 ) ) ;
#4846=ORIENTED_EDGE ( 'NONE', *, *, #13981, .F. ) ;
#4859=VECTOR ( 'NONE', #16547, 1000.000000000000000 ) ;
#4905=DIRECTION ( 'NONE',  ( 0.000000000000000000, 1.000000000000000000, -0.000000000000000000 ) ) ;
#4914=CARTESIAN_POINT ( 'NONE',  ( -79.54423376290921510, -91.42293805878655633, -41.30286037549884526 ) ) ;
#4940=FACE_OUTER_BOUND ( 'NONE', #15136, .T. ) ;
#4941=ORIENTED_EDGE ( 'NONE', *, *, #14634, .F. ) ;
#4974=CARTESIAN_POINT ( 'NONE',  ( -115.4692715616777434, -94.42547395655697073, 5.919112368231092880 ) ) ;
#4979=VERTEX_POINT ( 'NONE', #3341 ) ;
#5036=ADVANCED_FACE ( 'NONE', ( #4735 ), #9336, .F. ) ;
#5051=DIRECTION ( 'NONE',  ( 0.000000000000000000, 0.000000000000000000, 1.000000000000000000 ) ) ;
#5077=CIRCLE ( 'NONE', #16736, 5.000000000000000000 ) ;
#5086=ADVANCED_FACE ( 'NONE', ( #4940 ), #7835, .F. ) ;
#5095=VERTEX_POINT ( 'NONE', #10829 ) ;
#5100=( NAMED_UNIT ( * ) PLANE_ANGLE_UNIT ( ) SI_UNIT ( $, .RADIAN. ) );
#5119=ORIENTED_EDGE ( 'NONE', *, *, #8429, .T. ) ;
#5140=CARTESIAN_POINT ( 'NONE',  ( -27.58560781757364211, -92.35432432510553724, -7.309979984196388614 ) ) ;
#5146=EDGE_CURVE ( 'NONE', #13337, #12706, #6441, .T. ) ;
#5164=CARTESIAN_POINT ( 'NONE',  ( -112.3460510726627462, -91.53393135689864835, 8.561720054221641618 ) ) ;
#5169=VECTOR ( 'NONE', #10270, 1000.000000000000000 ) ;
#5177=DIRECTION ( 'NONE',  ( -0.000000000000000000, -1.000000000000000000, -0.000000000000000000 ) ) ;
#5187=AXIS2_PLACEMENT_3D ( 'NONE', #6310, #12322, #17740 ) ;
#5212=CARTESIAN_POINT ( 'NONE',  ( -65.06546592763127990, -111.0842361345572158, -2.621725226070001387E-13 ) ) ;
#5218=DIRECTION ( 'NONE',  ( 0.000000000000000000, 0.000000000000000000, -1.000000000000000000 ) ) ;
#5224=DIRECTION ( 'NONE',  ( -1.000000000000000000, -0.000000000000000000, -6.950654929607132427E-15 ) ) ;
#5277=CARTESIAN_POINT ( 'NONE',  ( -31.40585197410439378, -91.08930925317537231, 10.39386867823088068 ) ) ;
#5328=ORIENTED_EDGE ( 'NONE', *, *, #2403, .F. ) ;
#5332=CARTESIAN_POINT ( 'NONE',  ( -76.37409655828280108, -96.08423613455721579, 45.05044770573179846 ) ) ;
#5333=DIRECTION ( 'NONE',  ( 0.000000000000000000, 1.000000000000000000, -0.000000000000000000 ) ) ;
#5347=FACE_OUTER_BOUND ( 'NONE', #4304, .T. ) ;
#5353=CARTESIAN_POINT ( 'NONE',  ( -60.06546592763088910, -91.08423613455721579, -38.97384619189688948 ) ) ;
#5372=ORIENTED_EDGE ( 'NONE', *, *, #13609, .T. ) ;
#5412=DIRECTION ( 'NONE',  ( 1.047634945911800068E-14, -0.000000000000000000, -1.000000000000000000 ) ) ;
#5418=CARTESIAN_POINT ( 'NONE',  ( -81.37409655828280108, -91.08423613455721579, 38.97384619189696764 ) ) ;
#5420=DIRECTION ( 'NONE',  ( -0.000000000000000000, -1.000000000000000000, 0.000000000000000000 ) ) ;
#5430=DIRECTION ( 'NONE',  ( -0.000000000000000000, -1.000000000000000000, -0.000000000000000000 ) ) ;
#5453=CIRCLE ( 'NONE', #8459, 5.654315315325682434 ) ;
#5458=SHAPE_DEFINITION_REPRESENTATION ( #9535, #13055 ) ;
#5478=ADVANCED_FACE ( 'NONE', ( #16865 ), #2334, .T. ) ;
#5498=ADVANCED_FACE ( 'NONE', ( #5347 ), #2460, .T. ) ;
#5509=EDGE_CURVE ( 'NONE', #16233, #14058, #15272, .T. ) ;
#5512=CARTESIAN_POINT ( 'NONE',  ( -3.930119462002491844E-14, -91.08423613455721579, 5.654315315326165603 ) ) ;
#5515=CARTESIAN_POINT ( 'NONE',  ( -60.06546592763088910, -91.08423613455721579, -38.97384619189688948 ) ) ;
#5517=CIRCLE ( 'NONE', #1352, 5.000000000000004441 ) ;
#5530=CARTESIAN_POINT ( 'NONE',  ( -25.66933353722515676, -96.08423613455721579, -5.654315315325675328 ) ) ;
#5535=ORIENTED_EDGE ( 'NONE', *, *, #11354, .T. ) ;
#5549=ORIENTED_EDGE ( 'NONE', *, *, #7890, .F. ) ;
#5587=CARTESIAN_POINT ( 'NONE',  ( -25.66933353722515676, -91.08423613455721579, 5.654315315325685987 ) ) ;
#5597=ADVANCED_FACE ( 'NONE', ( #8061 ), #13692, .T. ) ;
#5604=FACE_OUTER_BOUND ( 'NONE', #14244, .T. ) ;
#5621=EDGE_CURVE ( 'NONE', #5840, #1115, #6001, .T. ) ;
#5634=AXIS2_PLACEMENT_3D ( 'NONE', #8732, #290, #17404 ) ;
#5636=CARTESIAN_POINT ( 'NONE',  ( -114.6525958062275095, -93.09900722835551790, -6.628862765693821046 ) ) ;
#5651=CARTESIAN_POINT ( 'NONE',  ( -70.71978124295708312, -111.0842361345572158, 28.18308811886538479 ) ) ;
#5657=AXIS2_PLACEMENT_3D ( 'NONE', #6799, #13918, #15496 ) ;
#5667=AXIS2_PLACEMENT_3D ( 'NONE', #17073, #14355, #15583 ) ;
#5670=ADVANCED_FACE ( 'NONE', ( #5818 ), #16982, .T. ) ;
#5683=VECTOR ( 'NONE', #17665, 1000.000000000000000 ) ;
#5685=VERTEX_POINT ( 'NONE', #662 ) ;
#5704=AXIS2_PLACEMENT_3D ( 'NONE', #16295, #17793, #17692 ) ;
#5719=CARTESIAN_POINT ( 'NONE',  ( -78.76908973550909820, -91.80660034481553566, 42.25011218277849423 ) ) ;
#5727=CARTESIAN_POINT ( 'NONE',  ( -109.6936274348538944, -91.08423613455721579, -10.65431531532595777 ) ) ;
#5743=FACE_OUTER_BOUND ( 'NONE', #9076, .T. ) ;
#5757=CIRCLE ( 'NONE', #9648, 10.65431531532568243 ) ;
#5781=CARTESIAN_POINT ( 'NONE',  ( 0.000000000000000000, 0.000000000000000000, 0.000000000000000000 ) ) ;
#5783=CARTESIAN_POINT ( 'NONE',  ( -60.58685171690446225, -91.10977296152348970, -39.65137083761668890 ) ) ;
#5799=AXIS2_PLACEMENT_3D ( 'NONE', #16995, #14613, #1712 ) ;
#5818=FACE_OUTER_BOUND ( 'NONE', #11934, .T. ) ;
#5838=ORIENTED_EDGE ( 'NONE', *, *, #10308, .T. ) ;
#5840=VERTEX_POINT ( 'NONE', #18358 ) ;
#5848=ORIENTED_EDGE ( 'NONE', *, *, #233, .T. ) ;
#5855=CARTESIAN_POINT ( 'NONE',  ( -31.74593505105995916, -91.08423613455721579, -10.65431531532567710 ) ) ;
#5865=ORIENTED_EDGE ( 'NONE', *, *, #9959, .F. ) ;
#5871=LINE ( 'NONE', #6128, #15012 ) ;
#5881=VERTEX_POINT ( 'NONE', #4041 ) ;
#5921=CARTESIAN_POINT ( 'NONE',  ( -76.37409655828236055, -111.0842361345572158, -28.18308811886544873 ) ) ;
#5939=EDGE_CURVE ( 'NONE', #513, #11655, #10418, .T. ) ;
#5951=CARTESIAN_POINT ( 'NONE',  ( -25.66933353722515676, -96.08423613455721579, 5.654315315325685987 ) ) ;
#5964=CARTESIAN_POINT ( 'NONE',  ( -25.66933353722515676, -91.08423613455721579, -5.654315315325675328 ) ) ;
#5980=CARTESIAN_POINT ( 'NONE',  ( -76.63889361118854993, -94.42547395655697073, 44.74949031872077398 ) ) ;
#5987=AXIS2_PLACEMENT_3D ( 'NONE', #7630, #4905, #13700 ) ;
#5990=DIRECTION ( 'NONE',  ( 0.000000000000000000, 1.000000000000000000, -0.000000000000000000 ) ) ;
#6001=B_SPLINE_CURVE_WITH_KNOTS ( 'NONE', 3,
 ( #13043, #121, #2744, #4237, #2930, #212, #5636, #7141, #12855, #8453, #8557, #11357, #17049, #3019, #1615, #10216, #9949, #24, #7403, #5727 ),
 .UNSPECIFIED., .F., .F.,
 ( 4, 2, 2, 2, 2, 2, 2, 2, 2, 4 ),
 ( 0.000000000000000000, 0.001278592738658804314, 0.002557185477317608629, 0.003835778215976412726, 0.005114370954635217258, 0.006392963693294019187, 0.007671556431952822851, 0.008950149170611624780, 0.009589445539941010566, 0.01022874190927039288 ),
 .UNSPECIFIED. ) ;
#6028=DIRECTION ( 'NONE',  ( 0.000000000000000000, 1.000000000000000000, -0.000000000000000000 ) ) ;
#6032=TOROIDAL_SURFACE ( 'NONE', #15000, 40.40389983439752086, 5.000000000000000000 ) ;
#6037=DIRECTION ( 'NONE',  ( 0.000000000000000000, 0.000000000000000000, 1.000000000000000000 ) ) ;
#6055=DIRECTION ( 'NONE',  ( -0.000000000000000000, -1.000000000000000000, -0.000000000000000000 ) ) ;
#6071=CARTESIAN_POINT ( 'NONE',  ( -60.06546592763127990, -96.08423613455721579, -2.420256967240809069E-13 ) ) ;
#6075=CARTESIAN_POINT ( 'NONE',  ( -76.42964172313227778, -95.23217669033336108, 44.98760873426157758 ) ) ;
#6084=CARTESIAN_POINT ( 'NONE',  ( -70.71978124295696944, -96.08423613455721579, 5.204170427930421283E-15 ) ) ;
#6086=LINE ( 'NONE', #2852, #9952 ) ;
#6088=CARTESIAN_POINT ( 'NONE',  ( -27.58560781757364211, -92.35432432510553724, 7.309979984196399272 ) ) ;
#6092=CARTESIAN_POINT ( 'NONE',  ( -60.06546592763129411, -96.08423613455721579, -6.292668114826103378E-13 ) ) ;
#6121=CARTESIAN_POINT ( 'NONE',  ( -42.53669312409158465, -91.08423613455721579, 5.204170427930421283E-15 ) ) ;
#6124=ORIENTED_EDGE ( 'NONE', *, *, #17608, .T. ) ;
#6128=CARTESIAN_POINT ( 'NONE',  ( -60.06546592763127990, -91.08423613455721579, -2.420256967240809069E-13 ) ) ;
#6143=EDGE_CURVE ( 'NONE', #2924, #3192, #4126, .T. ) ;
#6182=ADVANCED_FACE ( 'NONE', ( #2132 ), #4499, .T. ) ;
#6192=FACE_OUTER_BOUND ( 'NONE', #15828, .T. ) ;
#6198=ORIENTED_EDGE ( 'NONE', *, *, #17757, .T. ) ;
#6201=ORIENTED_EDGE ( 'NONE', *, *, #1942, .T. ) ;
#6210=EDGE_CURVE ( 'NONE', #5095, #10198, #7470, .T. ) ;
#6212=B_SPLINE_CURVE_WITH_KNOTS ( 'NONE', 3,
 ( #5515, #11240, #2904, #5783, #10096, #16925, #12748, #14393, #1408, #12646, #18344, #8419, #15624, #13008, #18435, #12817, #184, #4114, #9818, #14130 ),
 .UNSPECIFIED., .F., .F.,
 ( 4, 2, 2, 2, 2, 2, 2, 2, 2, 4 ),
 ( -1.439925654488655154E-05, 0.0006244272253376482703, 0.001263253707220183229, 0.002540906670985252497, 0.003818559634750321331, 0.005096212598515389297, 0.006373865562280459432, 0.007651518526045526965, 0.008929171489810596232, 0.01020682445357566463 ),
 .UNSPECIFIED. ) ;
#6216=DIRECTION ( 'NONE',  ( -4.029365176583844474E-15, 0.000000000000000000, 1.000000000000000000 ) ) ;
#6224=CARTESIAN_POINT ( 'NONE',  ( -70.71978124295696944, -96.08423613455721579, 5.204170427930421283E-15 ) ) ;
#6250=EDGE_LOOP ( 'NONE', ( #15771, #4042, #14803, #10765 ) ) ;
#6254=AXIS2_PLACEMENT_3D ( 'NONE', #16576, #12571, #3855 ) ;
#6261=CARTESIAN_POINT ( 'NONE',  ( -65.06546592763082515, -111.0842361345572158, -45.05044770573174873 ) ) ;
#6267=VERTEX_POINT ( 'NONE', #14383 ) ;
#6288=DIRECTION ( 'NONE',  ( 0.000000000000000000, 0.000000000000000000, 1.000000000000000000 ) ) ;
#6296=CARTESIAN_POINT ( 'NONE',  ( -65.06546592763082515, -96.08423613455721579, -45.05044770573174873 ) ) ;
#6300=ORIENTED_EDGE ( 'NONE', *, *, #16115, .T. ) ;
#6310=CARTESIAN_POINT ( 'NONE',  ( -70.71978124295708312, -91.08423613455721579, 28.18308811886538479 ) ) ;
#6324=ORIENTED_EDGE ( 'NONE', *, *, #10308, .F. ) ;
#6351=CARTESIAN_POINT ( 'NONE',  ( -31.40585197410439378, -91.08930925317537231, -10.39386867823087002 ) ) ;
#6361=CARTESIAN_POINT ( 'NONE',  ( -70.71978124295668522, -111.0842361345572158, -28.18308811886538479 ) ) ;
#6367=FACE_OUTER_BOUND ( 'NONE', #15451, .T. ) ;
#6389=AXIS2_PLACEMENT_3D ( 'NONE', #13334, #3049, #14469 ) ;
#6394=EDGE_CURVE ( 'NONE', #1115, #13953, #1398, .T. ) ;
#6417=DIRECTION ( 'NONE',  ( 0.000000000000000000, 1.000000000000000000, -0.000000000000000000 ) ) ;
#6441=B_SPLINE_CURVE_WITH_KNOTS ( 'NONE', 3,
 ( #13730, #18032, #13827, #15219, #9614, #11025, #3905, #10653, #2405, #1116, #15316, #1016, #12443, #18135, #16709, #16338, #8218, #6810, #3524, #9239 ),
 .UNSPECIFIED., .F., .F.,
 ( 4, 2, 2, 2, 2, 2, 2, 2, 2, 4 ),
 ( -1.439925654488133212E-05, 0.0006244272253376713638, 0.001263253707220224212, 0.002540906670985296299, 0.003818559634750368168, 0.005096212598515426594, 0.006373865562280486320, 0.007651518526045546914, 0.008929171489810606641, 0.01020682445357566810 ),
 .UNSPECIFIED. ) ;
#6458=DIRECTION ( 'NONE',  ( 0.000000000000000000, 1.000000000000000000, -0.000000000000000000 ) ) ;
#6462=CARTESIAN_POINT ( 'NONE',  ( 3.930119462001817841E-14, -91.08423613455721579, -5.654315315325195712 ) ) ;
#6477=ORIENTED_EDGE ( 'NONE', *, *, #9596, .F. ) ;
#6489=MANIFOLD_SOLID_BREP ( 'Fillet6', #17729 ) ;
#6491=LINE ( 'NONE', #3593, #11970 ) ;
#6501=( LENGTH_UNIT ( ) NAMED_UNIT ( * ) SI_UNIT ( .MILLI., .METRE. ) );
#6523=ADVANCED_FACE ( 'NONE', ( #5743 ), #8843, .T. ) ;
#6576=VECTOR ( 'NONE', #8432, 1000.000000000000000 ) ;
#6577=CYLINDRICAL_SURFACE ( 'NONE', #15271, 5.654315315325680658 ) ;
#6588=ORIENTED_EDGE ( 'NONE', *, *, #16115, .F. ) ;
#6591=CARTESIAN_POINT ( 'NONE',  ( -81.24478565583270040, -91.08423613455721579, -39.14322682088991456 ) ) ;
#6606=CARTESIAN_POINT ( 'NONE',  ( -65.06546592763146464, -111.0842361345572158, 45.05044770573184110 ) ) ;
#6644=CARTESIAN_POINT ( 'NONE',  ( -25.73217265163131984, -95.23217577251028843, -5.709860606646929071 ) ) ;
#6659=AXIS2_PLACEMENT_3D ( 'NONE', #6939, #13868, #12470 ) ;
#6662=ORIENTED_EDGE ( 'NONE', *, *, #10663, .T. ) ;
#6667=CARTESIAN_POINT ( 'NONE',  ( -115.7702289486887963, -95.65021661331553560, 5.654315315325360913 ) ) ;
#6674=AXIS2_PLACEMENT_3D ( 'NONE', #9595, #2490, #15299 ) ;
#6678=DIRECTION ( 'NONE',  ( -0.000000000000000000, -1.000000000000000000, -0.000000000000000000 ) ) ;
#6756=ADVANCED_FACE ( 'NONE', ( #6367 ), #9010, .T. ) ;
#6768=EDGE_CURVE ( 'NONE', #7404, #60, #17416, .T. ) ;
#6781=DIRECTION ( 'NONE',  ( -1.000000000000000000, 0.000000000000000000, -3.469446951953611033E-15 ) ) ;
#6799=CARTESIAN_POINT ( 'NONE',  ( -42.53669312409158465, -96.08423613455721579, -10.65431531532567533 ) ) ;
#6804=DIRECTION ( 'NONE',  ( 0.000000000000000000, 0.000000000000000000, 1.000000000000000000 ) ) ;
#6810=CARTESIAN_POINT ( 'NONE',  ( -65.00992063631021267, -95.23217577251026000, 44.98760859132568868 ) ) ;
#6817=ADVANCED_FACE ( 'NONE', ( #17592 ), #11725, .T. ) ;
#6833=EDGE_LOOP ( 'NONE', ( #11883, #1404, #7842, #6844 ) ) ;
#6844=ORIENTED_EDGE ( 'NONE', *, *, #13958, .F. ) ;
#6862=CARTESIAN_POINT ( 'NONE',  ( -81.37409655828237476, -91.08423613455721579, -28.18308811886549847 ) ) ;
#6877=CARTESIAN_POINT ( 'NONE',  ( -7.405446926806058452E-14, -91.08423613455721579, 10.65431531532616560 ) ) ;
#6939=CARTESIAN_POINT ( 'NONE',  ( -42.53669312409158465, -91.08423613455721579, 5.204170427930421283E-15 ) ) ;
#6991=EDGE_CURVE ( 'NONE', #3816, #17058, #17040, .T. ) ;
#6992=VECTOR ( 'NONE', #5412, 1000.000000000000000 ) ;
#7000=EDGE_CURVE ( 'NONE', #11655, #13953, #9603, .T. ) ;
#7068=ORIENTED_EDGE ( 'NONE', *, *, #18058, .F. ) ;
#7075=ORIENTED_EDGE ( 'NONE', *, *, #2430, .F. ) ;
#7080=ORIENTED_EDGE ( 'NONE', *, *, #11885, .T. ) ;
#7094=CARTESIAN_POINT ( 'NONE',  ( -76.37409655828236055, -96.08423613455721579, -28.18308811886544873 ) ) ;
#7114=CARTESIAN_POINT ( 'NONE',  ( -70.71978124295696944, -91.08423613455721579, 5.204170427930421283E-15 ) ) ;
#7117=ORIENTED_EDGE ( 'NONE', *, *, #13138, .F. ) ;
#7141=CARTESIAN_POINT ( 'NONE',  ( -114.1362093120868337, -92.58100082067039693, -7.070573948081583460 ) ) ;
#7176=APPLICATION_CONTEXT ( 'automotive_design' ) ;
#7245=CARTESIAN_POINT ( 'NONE',  ( -26.78696867915027724, -93.09900487505512956, 6.628864488196846594 ) ) ;
#7247=DIRECTION ( 'NONE',  ( -3.223492141267075737E-15, 0.000000000000000000, 1.000000000000000000 ) ) ;
#7252=CARTESIAN_POINT ( 'NONE',  ( 0.000000000000000000, -96.08423613455721579, -5.654315315325675328 ) ) ;
#7261=VERTEX_POINT ( 'NONE', #18131 ) ;
#7274=B_SPLINE_CURVE_WITH_KNOTS ( 'NONE', 3,
 ( #10307, #8633, #6075, #5980, #12946, #10388, #14337, #7588, #15825, #18, #5719, #7320, #1780, #1520, #208, #17139, #285, #13037, #4590, #11709 ),
 .UNSPECIFIED., .F., .F.,
 ( 4, 2, 2, 2, 2, 2, 2, 2, 2, 4 ),
 ( 0.000000000000000000, 0.001278592738658794990, 0.002557185477317589981, 0.003835778215976384971, 0.005114370954635179961, 0.006392963693293974084, 0.007671556431952769942, 0.008950149170611565799, 0.009589445539940970667, 0.01022874190927037553 ),
 .UNSPECIFIED. ) ;
#7320=CARTESIAN_POINT ( 'NONE',  ( -79.28150129717909067, -91.53393135689866256, 41.62626982970570566 ) ) ;
#7322=VERTEX_POINT ( 'NONE', #2606 ) ;
#7336=ORIENTED_EDGE ( 'NONE', *, *, #13609, .F. ) ;
#7385=PRODUCT_DEFINITION ( 'UNKNOWN', '', #10862, #15066 ) ;
#7403=CARTESIAN_POINT ( 'NONE',  ( -109.8630080638463511, -91.08423613455720158, -10.52500441287596011 ) ) ;
#7404=VERTEX_POINT ( 'NONE', #7094 ) ;
#7408=LINE ( 'NONE', #12962, #13275 ) ;
#7425=EDGE_CURVE ( 'NONE', #7647, #12706, #9021, .T. ) ;
#7448=ORIENTED_EDGE ( 'NONE', *, *, #15108, .T. ) ;
#7470=LINE ( 'NONE', #13189, #911 ) ;
#7475=EDGE_LOOP ( 'NONE', ( #5549, #3830, #2780, #5372 ) ) ;
#7482=FACE_OUTER_BOUND ( 'NONE', #15747, .T. ) ;
#7527=DIRECTION ( 'NONE',  ( -0.000000000000000000, -1.000000000000000000, 0.000000000000000000 ) ) ;
#7586=VERTEX_POINT ( 'NONE', #7801 ) ;
#7588=CARTESIAN_POINT ( 'NONE',  ( -77.79035519103837260, -92.58100082067043957, 43.41642806912991404 ) ) ;
#7602=CARTESIAN_POINT ( 'NONE',  ( -42.53669312409158465, -91.08423613455721579, -5.654315315325675328 ) ) ;
#7624=DIRECTION ( 'NONE',  ( 0.000000000000000000, 1.000000000000000000, -0.000000000000000000 ) ) ;
#7630=CARTESIAN_POINT ( 'NONE',  ( 0.000000000000000000, -91.08423613455721579, 0.000000000000000000 ) ) ;
#7643=EDGE_CURVE ( 'NONE', #4979, #9931, #10504, .T. ) ;
#7647=VERTEX_POINT ( 'NONE', #13331 ) ;
#7657=ADVANCED_FACE ( 'NONE', ( #6192 ), #6032, .T. ) ;
#7691=ADVANCED_BREP_SHAPE_REPRESENTATION ( '', ( #6489, #16217 ), #17131 ) ;
#7696=VERTEX_POINT ( 'NONE', #5353 ) ;
#7714=CARTESIAN_POINT ( 'NONE',  ( -70.71978124295696944, -111.0842361345572158, 5.204170427930421283E-15 ) ) ;
#7716=CARTESIAN_POINT ( 'NONE',  ( -76.37409655828219002, -96.08423613455721579, -45.05044770573186952 ) ) ;
#7748=CARTESIAN_POINT ( 'NONE',  ( -76.37409655828265898, -111.0842361345572158, -8.001217251689905290E-13 ) ) ;
#7752=LINE ( 'NONE', #12069, #5683 ) ;
#7801=CARTESIAN_POINT ( 'NONE',  ( -115.7702289486888247, -96.08423613455721579, 5.654315315325360913 ) ) ;
#7804=AXIS2_PLACEMENT_3D ( 'NONE', #4530, #7527, #10074 ) ;
#7809=DIRECTION ( 'NONE',  ( -4.163336342344339393E-15, 0.000000000000000000, 1.000000000000000000 ) ) ;
#7835=PLANE ( 'NONE',  #11081 ) ;
#7842=ORIENTED_EDGE ( 'NONE', *, *, #17726, .T. ) ;
#7863=EDGE_CURVE ( 'NONE', #4718, #16572, #12653, .T. ) ;
#7872=VERTEX_POINT ( 'NONE', #6862 ) ;
#7877=ORIENTED_EDGE ( 'NONE', *, *, #4350, .F. ) ;
#7879=FACE_OUTER_BOUND ( 'NONE', #13709, .T. ) ;
#7881=CARTESIAN_POINT ( 'NONE',  ( -111.0396820472914214, -91.18731257919067446, 9.610190611755312418 ) ) ;
#7890=EDGE_CURVE ( 'NONE', #11836, #5685, #6086, .T. ) ;
#7913=CARTESIAN_POINT ( 'NONE',  ( -80.06812138002644019, -91.24992890033503556, -40.65007677557141363 ) ) ;
#7918=EDGE_CURVE ( 'NONE', #11153, #15074, #398, .T. ) ;
#7936=VERTEX_POINT ( 'NONE', #8561 ) ;
#7952=ORIENTED_EDGE ( 'NONE', *, *, #17757, .F. ) ;
#7957=CARTESIAN_POINT ( 'NONE',  ( -28.16748190072492974, -91.96845925178433845, -7.798233810088249562 ) ) ;
#7958=CARTESIAN_POINT ( 'NONE',  ( -98.90286936182235422, -96.08423613455721579, -2.027180301682503564E-13 ) ) ;
#7966=EDGE_LOOP ( 'NONE', ( #3380, #5119, #3833, #9811 ) ) ;
#7970=CARTESIAN_POINT ( 'NONE',  ( -113.2720846013049822, -91.96846159163192169, 7.798230460770113837 ) ) ;
#7979=DIRECTION ( 'NONE',  ( 0.000000000000000000, 0.000000000000000000, 1.000000000000000000 ) ) ;
#7994=CARTESIAN_POINT ( 'NONE',  ( -80.72210053294847398, -91.12516209206945916, -39.81919198398661308 ) ) ;
#7995=ORIENTED_EDGE ( 'NONE', *, *, #3608, .T. ) ;
#8006=ORIENTED_EDGE ( 'NONE', *, *, #10063, .F. ) ;
#8012=AXIS2_PLACEMENT_3D ( 'NONE', #10125, #2061, #17779 ) ;
#8035=DIRECTION ( 'NONE',  ( 0.000000000000000000, 0.000000000000000000, 1.000000000000000000 ) ) ;
#8061=FACE_OUTER_BOUND ( 'NONE', #14728, .T. ) ;
#8108=EDGE_CURVE ( 'NONE', #13982, #4718, #5757, .T. ) ;
#8125=VECTOR ( 'NONE', #10848, 1000.000000000000000 ) ;
#8135=ORIENTED_EDGE ( 'NONE', *, *, #7863, .T. ) ;
#8142=CARTESIAN_POINT ( 'NONE',  ( -30.39988730823796104, -91.18731141006421126, -9.610196039195443518 ) ) ;
#8146=ORIENTED_EDGE ( 'NONE', *, *, #14960, .T. ) ;
#8184=CARTESIAN_POINT ( 'NONE',  ( -70.71978124295668522, -96.08423613455721579, -28.18308811886538479 ) ) ;
#8186=AXIS2_PLACEMENT_3D ( 'NONE', #6361, #6458, #10592 ) ;
#8218=CARTESIAN_POINT ( 'NONE',  ( -64.80066835027112404, -94.42547236494611695, 44.74948972093436339 ) ) ;
#8337=EDGE_CURVE ( 'NONE', #16250, #13337, #5871, .T. ) ;
#8415=MECHANICAL_DESIGN_GEOMETRIC_PRESENTATION_REPRESENTATION('',(#8709),#2738);
#8419=CARTESIAN_POINT ( 'NONE',  ( -63.40980125876012607, -92.35432432510548040, -43.13417342538324561 ) ) ;
#8429=EDGE_CURVE ( 'NONE', #9931, #7647, #13090, .T. ) ;
#8432=DIRECTION ( 'NONE',  ( -0.000000000000000000, -1.000000000000000000, -0.000000000000000000 ) ) ;
#8448=VECTOR ( 'NONE', #2373, 1000.000000000000000 ) ;
#8453=CARTESIAN_POINT ( 'NONE',  ( -113.2720846013048543, -91.96846159163189327, -7.798230460770719574 ) ) ;
#8459=AXIS2_PLACEMENT_3D ( 'NONE', #8184, #11472, #11375 ) ;
#8532=EDGE_LOOP ( 'NONE', ( #516, #467, #16941, #14641, #10830 ) ) ;
#8544=FACE_OUTER_BOUND ( 'NONE', #15729, .T. ) ;
#8547=CARTESIAN_POINT ( 'NONE',  ( -65.06546592763129411, -111.0842361345572158, -6.816485587782003001E-13 ) ) ;
#8557=CARTESIAN_POINT ( 'NONE',  ( -112.9698934257354352, -91.80660034481556409, -8.049308492552277983 ) ) ;
#8561=CARTESIAN_POINT ( 'NONE',  ( -65.06546592763139358, -111.0842361345572158, 28.18308811886540610 ) ) ;
#8621=ORIENTED_EDGE ( 'NONE', *, *, #3608, .F. ) ;
#8633=CARTESIAN_POINT ( 'NONE',  ( -76.37409655828278687, -95.65021661331557823, 45.05044770573179846 ) ) ;
#8636=ORIENTED_EDGE ( 'NONE', *, *, #13387, .F. ) ;
#8673=CARTESIAN_POINT ( 'NONE',  ( -81.37409655828275845, -91.08423613455721579, 28.18308811886534571 ) ) ;
#8679=ORIENTED_EDGE ( 'NONE', *, *, #5146, .T. ) ;
#8704=EDGE_CURVE ( 'NONE', #4718, #7872, #9302, .T. ) ;
#8709=STYLED_ITEM('',(#18545),#6489);
#8715=VECTOR ( 'NONE', #3663, 1000.000000000000000 ) ;
#8726=AXIS2_PLACEMENT_3D ( 'NONE', #1518, #15546, #11539 ) ;
#8732=CARTESIAN_POINT ( 'NONE',  ( -98.90286936182235422, -96.08423613455721579, -2.027180301682503564E-13 ) ) ;
#8744=ORIENTED_EDGE ( 'NONE', *, *, #11258, .F. ) ;
#8755=AXIS2_PLACEMENT_3D ( 'NONE', #13403, #582, #9381 ) ;
#8778=ORIENTED_EDGE ( 'NONE', *, *, #8429, .F. ) ;
#8799=LINE ( 'NONE', #5964, #3012 ) ;
#8801=ORIENTED_EDGE ( 'NONE', *, *, #8108, .T. ) ;
#8811=DIRECTION ( 'NONE',  ( 0.000000000000000000, 0.000000000000000000, 1.000000000000000000 ) ) ;
#8813=CARTESIAN_POINT ( 'NONE',  ( -76.37409655828275845, -111.0842361345572158, 28.18308811886536347 ) ) ;
#8823=ADVANCED_FACE ( 'NONE', ( #2364 ), #6577, .F. ) ;
#8827=CIRCLE ( 'NONE', #13308, 5.654315315325682434 ) ;
#8832=EDGE_CURVE ( 'NONE', #2924, #13982, #3616, .T. ) ;
#8840=LINE ( 'NONE', #7602, #8715 ) ;
#8843=CYLINDRICAL_SURFACE ( 'NONE', #9901, 5.000000000000004441 ) ;
#8856=EDGE_LOOP ( 'NONE', ( #614, #16845, #9417, #13974 ) ) ;
#8860=CARTESIAN_POINT ( 'NONE',  ( -76.37409655828265898, -91.08423613455721579, -2.461913000519969422E-13 ) ) ;
#8865=ORIENTED_EDGE ( 'NONE', *, *, #6394, .F. ) ;
#8919=PLANE ( 'NONE',  #12438 ) ;
#8948=AXIS2_PLACEMENT_3D ( 'NONE', #15009, #2379, #15110 ) ;
#8961=DIRECTION ( 'NONE',  ( 1.000000000000000000, 0.000000000000000000, 0.000000000000000000 ) ) ;
#8975=B_SPLINE_CURVE_WITH_KNOTS ( 'NONE', 3,
 ( #7716, #4810, #2202, #12031, #9415, #17730, #12212, #10529, #3413, #9135, #2289, #3705, #4914, #7913, #2013, #7994, #13428, #888, #6591, #10631 ),
 .UNSPECIFIED., .F., .F.,
 ( 4, 2, 2, 2, 2, 2, 2, 2, 2, 4 ),
 ( 0.000000000000000000, 0.001278592738658801062, 0.002557185477317602124, 0.003835778215976403185, 0.005114370954635204247, 0.006392963693294006176, 0.007671556431952806371, 0.008950149170611607433, 0.009589445539941000157, 0.01022874190927039288 ),
 .UNSPECIFIED. ) ;
#9009=ORIENTED_EDGE ( 'NONE', *, *, #14812, .F. ) ;
#9010=CYLINDRICAL_SURFACE ( 'NONE', #5704, 5.000000000000000000 ) ;
#9021=CIRCLE ( 'NONE', #15292, 45.40389983439752086 ) ;
#9029=CARTESIAN_POINT ( 'NONE',  ( -81.37409655828226107, -91.08423613455721579, -38.97384619189710975 ) ) ;
#9031=EDGE_CURVE ( 'NONE', #7261, #7647, #3602, .T. ) ;
#9034=EDGE_CURVE ( 'NONE', #4979, #7322, #8840, .T. ) ;
#9076=EDGE_LOOP ( 'NONE', ( #16411, #10232, #18286, #15065 ) ) ;
#9087=LINE ( 'NONE', #480, #4859 ) ;
#9096=CIRCLE ( 'NONE', #8186, 5.654315315325682434 ) ;
#9109=CARTESIAN_POINT ( 'NONE',  ( -111.3698580185283760, -91.24992890033504978, 9.348340137069554245 ) ) ;
#9123=DIRECTION ( 'NONE',  ( 1.110223024625157172E-14, -6.938893903907068633E-16, -1.000000000000000000 ) ) ;
#9127=DIRECTION ( 'NONE',  ( 1.000000000000000000, 0.000000000000000000, 4.163336342344339393E-15 ) ) ;
#9133=AXIS2_PLACEMENT_3D ( 'NONE', #9331, #16702, #6804 ) ;
#9134=DIRECTION ( 'NONE',  ( 0.000000000000000000, 0.000000000000000000, 1.000000000000000000 ) ) ;
#9135=CARTESIAN_POINT ( 'NONE',  ( -78.51801170372698380, -91.96846159163195011, -42.55230335834804833 ) ) ;
#9154=LINE ( 'NONE', #5212, #17095 ) ;
#9183=DIRECTION ( 'NONE',  ( 0.000000000000000000, 1.000000000000000000, -0.000000000000000000 ) ) ;
#9211=LINE ( 'NONE', #3692, #2527 ) ;
#9216=LINE ( 'NONE', #2009, #16502 ) ;
#9218=ORIENTED_EDGE ( 'NONE', *, *, #11258, .T. ) ;
#9239=CARTESIAN_POINT ( 'NONE',  ( -65.06546592763146464, -96.08423613455721579, 45.05044770573184110 ) ) ;
#9296=ORIENTED_EDGE ( 'NONE', *, *, #4350, .T. ) ;
#9297=ORIENTED_EDGE ( 'NONE', *, *, #14267, .T. ) ;
#9302=CIRCLE ( 'NONE', #7804, 10.65431531532568243 ) ;
#9309=CARTESIAN_POINT ( 'NONE',  ( 0.000000000000000000, -91.08423613455721579, 5.654315315325685987 ) ) ;
#9313=DIRECTION ( 'NONE',  ( -1.000000000000000000, 0.000000000000000000, 0.000000000000000000 ) ) ;
#9320=EDGE_CURVE ( 'NONE', #17849, #3192, #14593, .T. ) ;
#9331=CARTESIAN_POINT ( 'NONE',  ( -70.71978124295668522, -96.08423613455721579, -28.18308811886538479 ) ) ;
#9336=CYLINDRICAL_SURFACE ( 'NONE', #17329, 5.654315315325682434 ) ;
#9359=VECTOR ( 'NONE', #5224, 1000.000000000000000 ) ;
#9362=CARTESIAN_POINT ( 'NONE',  ( -30.06971094502080177, -91.24992749556385263, -9.348345296714480668 ) ) ;
#9373=DIRECTION ( 'NONE',  ( -1.000000000000000000, 0.000000000000000000, -6.950654929607132427E-15 ) ) ;
#9381=DIRECTION ( 'NONE',  ( -6.950654929607131638E-15, 0.000000000000000000, 1.000000000000000000 ) ) ;
#9396=EDGE_CURVE ( 'NONE', #7586, #16233, #15052, .T. ) ;
#9415=CARTESIAN_POINT ( 'NONE',  ( -76.78641432137852973, -94.06000857856476216, -44.58117269483251022 ) ) ;
#9417=ORIENTED_EDGE ( 'NONE', *, *, #6210, .T. ) ;
#9443=ORIENTED_EDGE ( 'NONE', *, *, #4024, .F. ) ;
#9455=CARTESIAN_POINT ( 'NONE',  ( -26.13860949178274851, -94.06000665574431707, -6.066633903742957301 ) ) ;
#9479=EDGE_LOOP ( 'NONE', ( #11385, #3787, #14953, #15173 ) ) ;
#9480=PRODUCT_CONTEXT ( 'NONE', #3453, 'mechanical' ) ;
#9505=CARTESIAN_POINT ( 'NONE',  ( -76.37409655828265898, -96.08423613455721579, -8.001217251689905290E-13 ) ) ;
#9512=AXIS2_PLACEMENT_3D ( 'NONE', #7958, #17957, #13669 ) ;
#9518=DIRECTION ( 'NONE',  ( 1.047634945911799279E-14, 0.000000000000000000, -1.000000000000000000 ) ) ;
#9535=PRODUCT_DEFINITION_SHAPE ( 'NONE', 'NONE',  #7385 ) ;
#9552=FACE_OUTER_BOUND ( 'NONE', #10535, .T. ) ;
#9578=( NAMED_UNIT ( * ) PLANE_ANGLE_UNIT ( ) SI_UNIT ( $, .RADIAN. ) );
#9595=CARTESIAN_POINT ( 'NONE',  ( -42.53669312409158465, -111.0842361345572158, 5.204170427930421283E-15 ) ) ;
#9596=EDGE_CURVE ( 'NONE', #800, #7936, #11142, .T. ) ;
#9603=CIRCLE ( 'NONE', #8726, 5.000000000000000000 ) ;
#9614=CARTESIAN_POINT ( 'NONE',  ( -60.71745612804077297, -91.12516132330414109, 39.81918451580458651 ) ) ;
#9626=EDGE_CURVE ( 'NONE', #7586, #513, #1325, .T. ) ;
#9641=CIRCLE ( 'NONE', #10238, 45.40389983439752086 ) ;
#9643=AXIS2_PLACEMENT_3D ( 'NONE', #16025, #14802, #15166 ) ;
#9648=AXIS2_PLACEMENT_3D ( 'NONE', #4686, #2161, #16466 ) ;
#9649=FACE_OUTER_BOUND ( 'NONE', #3392, .T. ) ;
#9655=AXIS2_PLACEMENT_3D ( 'NONE', #3190, #117, #11805 ) ;
#9667=DIRECTION ( 'NONE',  ( 0.000000000000000000, 0.000000000000000000, 1.000000000000000000 ) ) ;
#9670=VECTOR ( 'NONE', #3825, 1000.000000000000000 ) ;
#9675=DIRECTION ( 'NONE',  ( -1.000000000000000000, 0.000000000000000000, 0.000000000000000000 ) ) ;
#9698=AXIS2_PLACEMENT_3D ( 'NONE', #8860, #1732, #13150 ) ;
#9721=EDGE_CURVE ( 'NONE', #7261, #17089, #2531, .T. ) ;
#9725=VERTEX_POINT ( 'NONE', #5418 ) ;
#9731=DIRECTION ( 'NONE',  ( -1.000000000000000000, 0.000000000000000000, -6.950654929607132427E-15 ) ) ;
#9738=CARTESIAN_POINT ( 'NONE',  ( -3.930119462002491844E-14, -96.08423613455721579, 5.654315315326165603 ) ) ;
#9774=ORIENTED_EDGE ( 'NONE', *, *, #2145, .F. ) ;
#9793=ORIENTED_EDGE ( 'NONE', *, *, #4684, .T. ) ;
#9811=ORIENTED_EDGE ( 'NONE', *, *, #14757, .T. ) ;
#9818=CARTESIAN_POINT ( 'NONE',  ( -65.06546592763085357, -95.65021616327642562, -45.05044770573176294 ) ) ;
#9836=DIRECTION ( 'NONE',  ( 0.000000000000000000, 0.000000000000000000, -1.000000000000000000 ) ) ;
#9844=CIRCLE ( 'NONE', #14324, 10.65431531532567888 ) ;
#9901=AXIS2_PLACEMENT_3D ( 'NONE', #221, #7247, #17324 ) ;
#9920=VECTOR ( 'NONE', #17135, 1000.000000000000000 ) ;
#9926=ORIENTED_EDGE ( 'NONE', *, *, #7000, .F. ) ;
#9929=CARTESIAN_POINT ( 'NONE',  ( -65.06546592763099568, -91.08423613455721579, -28.18308811886532084 ) ) ;
#9931=VERTEX_POINT ( 'NONE', #11773 ) ;
#9933=EDGE_LOOP ( 'NONE', ( #15707, #11724, #11743, #6662 ) ) ;
#9949=CARTESIAN_POINT ( 'NONE',  ( -110.3711597500467860, -91.10977358899565104, -10.13292356933350113 ) ) ;
#9952=VECTOR ( 'NONE', #4509, 1000.000000000000000 ) ;
#9959=EDGE_CURVE ( 'NONE', #11836, #7586, #10226, .T. ) ;
#9972=ORIENTED_EDGE ( 'NONE', *, *, #6143, .F. ) ;
#9974=CIRCLE ( 'NONE', #9655, 45.40389983439752086 ) ;
#9996=DIRECTION ( 'NONE',  ( 2.750867011994134873E-15, 0.000000000000000000, 1.000000000000000000 ) ) ;
#10039=ORIENTED_EDGE ( 'NONE', *, *, #16467, .F. ) ;
#10053=CARTESIAN_POINT ( 'NONE',  ( -26.13860949178274851, -94.06000665574431707, 6.066633903742967071 ) ) ;
#10063=EDGE_CURVE ( 'NONE', #16572, #2924, #5453, .T. ) ;
#10074=DIRECTION ( 'NONE',  ( 0.000000000000000000, 0.000000000000000000, 1.000000000000000000 ) ) ;
#10096=CARTESIAN_POINT ( 'NONE',  ( -60.71745612804021874, -91.12516132330414109, -39.81918451580444440 ) ) ;
#10125=CARTESIAN_POINT ( 'NONE',  ( -70.71978124295708312, -96.08423613455721579, 28.18308811886538479 ) ) ;
#10153=CIRCLE ( 'NONE', #6254, 40.40389983439752086 ) ;
#10198=VERTEX_POINT ( 'NONE', #3033 ) ;
#10213=AXIS2_PLACEMENT_3D ( 'NONE', #18266, #15077, #17116 ) ;
#10216=CARTESIAN_POINT ( 'NONE',  ( -110.5389732269433978, -91.12516209206943074, -10.00231928999220621 ) ) ;
#10226=CIRCLE ( 'NONE', #12643, 45.40389983439752086 ) ;
#10232=ORIENTED_EDGE ( 'NONE', *, *, #642, .F. ) ;
#10238=AXIS2_PLACEMENT_3D ( 'NONE', #12378, #853, #5051 ) ;
#10262=ADVANCED_FACE ( 'NONE', ( #1713 ), #10332, .T. ) ;
#10270=DIRECTION ( 'NONE',  ( 1.000000000000000000, -0.000000000000000000, -0.000000000000000000 ) ) ;
#10280=VECTOR ( 'NONE', #17829, 1000.000000000000000 ) ;
#10288=TOROIDAL_SURFACE ( 'NONE', #18370, 10.65431531532568243, 5.000000000000000000 ) ;
#10307=CARTESIAN_POINT ( 'NONE',  ( -76.37409655828280108, -96.08423613455721579, 45.05044770573179846 ) ) ;
#10308=EDGE_CURVE ( 'NONE', #7586, #5881, #16424, .T. ) ;
#10318=ADVANCED_FACE ( 'NONE', ( #14978 ), #16298, .T. ) ;
#10332=CYLINDRICAL_SURFACE ( 'NONE', #9643, 45.40389983439752086 ) ;
#10388=CARTESIAN_POINT ( 'NONE',  ( -77.14491745292085056, -93.39009998357852282, 44.16867553823936277 ) ) ;
#10408=CARTESIAN_POINT ( 'NONE',  ( -65.06546592763127990, -91.08423613455721579, -2.621725226070001387E-13 ) ) ;
#10418=CIRCLE ( 'NONE', #9512, 5.654315315325680658 ) ;
#10435=AXIS2_PLACEMENT_3D ( 'NONE', #6121, #14478, #1567 ) ;
#10471=FACE_OUTER_BOUND ( 'NONE', #247, .T. ) ;
#10503=ORIENTED_EDGE ( 'NONE', *, *, #18058, .T. ) ;
#10504=CIRCLE ( 'NONE', #14989, 5.654315315325680658 ) ;
#10528=EDGE_CURVE ( 'NONE', #11836, #9725, #7274, .T. ) ;
#10529=CARTESIAN_POINT ( 'NONE',  ( -77.79035519103784679, -92.58100082067039693, -43.41642806912999930 ) ) ;
#10535=EDGE_LOOP ( 'NONE', ( #14458, #1351, #7448, #11401 ) ) ;
#10551=DIRECTION ( 'NONE',  ( 0.000000000000000000, 0.000000000000000000, 1.000000000000000000 ) ) ;
#10569=CARTESIAN_POINT ( 'NONE',  ( -25.66933353722515676, -111.0842361345572158, 5.654315315325685987 ) ) ;
#10577=EDGE_CURVE ( 'NONE', #10198, #3816, #9974, .T. ) ;
#10586=CIRCLE ( 'NONE', #5799, 5.654315315325680658 ) ;
#10592=DIRECTION ( 'NONE',  ( 0.000000000000000000, 0.000000000000000000, 1.000000000000000000 ) ) ;
#10604=CARTESIAN_POINT ( 'NONE',  ( -109.6936274348540508, -91.08423613455721579, 10.65431531532540177 ) ) ;
#10612=CIRCLE ( 'NONE', #17190, 5.654315315325682434 ) ;
#10631=CARTESIAN_POINT ( 'NONE',  ( -81.37409655828226107, -91.08423613455721579, -38.97384619189710975 ) ) ;
#10653=CARTESIAN_POINT ( 'NONE',  ( -61.89532410461230683, -91.42293623445493722, 41.30285466933285221 ) ) ;
#10661=CARTESIAN_POINT ( 'NONE',  ( -115.7702289486887395, -96.08423613455721579, -5.654315315326000402 ) ) ;
#10663=EDGE_CURVE ( 'NONE', #5685, #15472, #9087, .T. ) ;
#10664=DIRECTION ( 'NONE',  ( -1.047634945911800068E-14, 0.000000000000000000, 1.000000000000000000 ) ) ;
#10685=CARTESIAN_POINT ( 'NONE',  ( -76.37409655828236055, -91.08423613455721579, -28.18308811886544873 ) ) ;
#10688=CARTESIAN_POINT ( 'NONE',  ( -110.5389732269435115, -91.12516209206941653, 10.00231928999164133 ) ) ;
#10696=ADVANCED_FACE ( 'NONE', ( #16637 ), #11750, .T. ) ;
#10765=ORIENTED_EDGE ( 'NONE', *, *, #5509, .F. ) ;
#10781=CARTESIAN_POINT ( 'NONE',  ( -114.6525958062276231, -93.09900722835551790, 6.628862765693201098 ) ) ;
#10791=CARTESIAN_POINT ( 'NONE',  ( -70.71978124295708312, -91.08423613455721579, 22.52877280353970235 ) ) ;
#10829=CARTESIAN_POINT ( 'NONE',  ( -76.37409655828219002, -96.08423613455721579, -45.05044770573186952 ) ) ;
#10830=ORIENTED_EDGE ( 'NONE', *, *, #3164, .F. ) ;
#10843=CARTESIAN_POINT ( 'NONE',  ( -81.37409655828265898, -91.08423613455721579, -8.525034724645805924E-13 ) ) ;
#10848=DIRECTION ( 'NONE',  ( 1.000000000000000000, 0.000000000000000000, 6.950654929607132427E-15 ) ) ;
#10857=CARTESIAN_POINT ( 'NONE',  ( -27.30335599338096841, -92.58099833983887095, -7.070576347711321930 ) ) ;
#10862=PRODUCT_DEFINITION_FORMATION_WITH_SPECIFIED_SOURCE ( 'ANY', '', #18381, .NOT_KNOWN. ) ;
#10873=ADVANCED_FACE ( 'NONE', ( #14829 ), #620, .F. ) ;
#10875=DIRECTION ( 'NONE',  ( -0.000000000000000000, -1.000000000000000000, -0.000000000000000000 ) ) ;
#10879=CARTESIAN_POINT ( 'NONE',  ( -110.3711597500469566, -91.10977358899566525, 10.13292356933293270 ) ) ;
#10902=CARTESIAN_POINT ( 'NONE',  ( -98.90286936182235422, -91.08423613455721579, -2.027180301682503564E-13 ) ) ;
#10937=DIRECTION ( 'NONE',  ( 1.000000000000000000, -0.000000000000000000, 1.047634945911799279E-14 ) ) ;
#10957=CARTESIAN_POINT ( 'NONE',  ( -30.90059672715241845, -91.12516132330414109, -10.00232511491633325 ) ) ;
#10976=DIRECTION ( 'NONE',  ( 0.000000000000000000, 1.000000000000000000, -0.000000000000000000 ) ) ;
#10985=ORIENTED_EDGE ( 'NONE', *, *, #9034, .T. ) ;
#10988=EDGE_CURVE ( 'NONE', #7322, #14963, #2820, .T. ) ;
#10989=CARTESIAN_POINT ( 'NONE',  ( -31.06841040534018106, -91.10977296152353233, 10.13292952605207375 ) ) ;
#11025=CARTESIAN_POINT ( 'NONE',  ( -61.10958520376166803, -91.18731141006419705, 40.31989393471906169 ) ) ;
#11030=CIRCLE ( 'NONE', #5657, 4.999999999999999112 ) ;
#11053=DIRECTION ( 'NONE',  ( 0.000000000000000000, 0.000000000000000000, 1.000000000000000000 ) ) ;
#11058=VECTOR ( 'NONE', #1385, 1000.000000000000000 ) ;
#11067=VERTEX_POINT ( 'NONE', #1647 ) ;
#11080=CARTESIAN_POINT ( 'NONE',  ( -30.90059672715241845, -91.12516132330414109, 10.00232511491634568 ) ) ;
#11081=AXIS2_PLACEMENT_3D ( 'NONE', #13550, #10937, #9518 ) ;
#11083=DIRECTION ( 'NONE',  ( -0.000000000000000000, -1.000000000000000000, -0.000000000000000000 ) ) ;
#11086=CARTESIAN_POINT ( 'NONE',  ( -98.90286936182231159, -91.08423613455721579, -5.654315315325883162 ) ) ;
#11113=ORIENTED_EDGE ( 'NONE', *, *, #12022, .T. ) ;
#11142=LINE ( 'NONE', #3745, #12011 ) ;
#11153=VERTEX_POINT ( 'NONE', #3144 ) ;
#11160=AXIS2_PLACEMENT_3D ( 'NONE', #15361, #5333, #11053 ) ;
#11203=CIRCLE ( 'NONE', #6389, 5.000000000000000888 ) ;
#11214=AXIS2_PLACEMENT_3D ( 'NONE', #6084, #5990, #1891 ) ;
#11240=CARTESIAN_POINT ( 'NONE',  ( -60.19468178563322169, -91.08423613455723000, -39.14310232490480956 ) ) ;
#11245=EDGE_CURVE ( 'NONE', #513, #14058, #836, .T. ) ;
#11246=CARTESIAN_POINT ( 'NONE',  ( -76.37409655828265898, -91.08423613455721579, -8.001217251689905290E-13 ) ) ;
#11258=EDGE_CURVE ( 'NONE', #7872, #3710, #13658, .T. ) ;
#11259=ORIENTED_EDGE ( 'NONE', *, *, #13138, .T. ) ;
#11274=ORIENTED_EDGE ( 'NONE', *, *, #3420, .F. ) ;
#11326=PLANE ( 'NONE',  #15080 ) ;
#11354=EDGE_CURVE ( 'NONE', #7696, #16406, #6212, .T. ) ;
#11357=CARTESIAN_POINT ( 'NONE',  ( -112.3460510726626040, -91.53393135689863414, -8.561720054222236698 ) ) ;
#11361=ORIENTED_EDGE ( 'NONE', *, *, #9320, .T. ) ;
#11375=DIRECTION ( 'NONE',  ( 0.000000000000000000, 0.000000000000000000, 1.000000000000000000 ) ) ;
#11385=ORIENTED_EDGE ( 'NONE', *, *, #12147, .F. ) ;
#11401=ORIENTED_EDGE ( 'NONE', *, *, #6991, .T. ) ;
#11408=DIRECTION ( 'NONE',  ( 1.000000000000000000, 0.000000000000000000, 6.950654929607132427E-15 ) ) ;
#11420=DIRECTION ( 'NONE',  ( 0.000000000000000000, 0.000000000000000000, -1.000000000000000000 ) ) ;
#11441=ORIENTED_EDGE ( 'NONE', *, *, #12137, .T. ) ;
#11464=CARTESIAN_POINT ( 'NONE',  ( -26.55110732739451507, -93.39009773859100960, 6.425137615056152995 ) ) ;
#11472=DIRECTION ( 'NONE',  ( 0.000000000000000000, 1.000000000000000000, -0.000000000000000000 ) ) ;
#11508=CARTESIAN_POINT ( 'NONE',  ( -70.71978124295696944, -96.08423613455721579, 5.204170427930421283E-15 ) ) ;
#11515=CIRCLE ( 'NONE', #15688, 45.40389983439752086 ) ;
#11517=AXIS2_PLACEMENT_3D ( 'NONE', #12867, #39, #6781 ) ;
#11539=DIRECTION ( 'NONE',  ( -8.326672684688674053E-15, 0.000000000000000000, 1.000000000000000000 ) ) ;
#11587=EDGE_CURVE ( 'NONE', #9725, #13598, #13542, .T. ) ;
#11630=DIRECTION ( 'NONE',  ( -4.029365176583844474E-15, 0.000000000000000000, 1.000000000000000000 ) ) ;
#11651=CARTESIAN_POINT ( 'NONE',  ( -115.7702289486888247, -111.0842361345572158, 5.654315315325360913 ) ) ;
#11655=VERTEX_POINT ( 'NONE', #13920 ) ;
#11709=CARTESIAN_POINT ( 'NONE',  ( -81.37409655828280108, -91.08423613455721579, 38.97384619189696764 ) ) ;
#11721=ORIENTED_EDGE ( 'NONE', *, *, #16007, .T. ) ;
#11724=ORIENTED_EDGE ( 'NONE', *, *, #642, .T. ) ;
#11725=CYLINDRICAL_SURFACE ( 'NONE', #17657, 45.40389983439752086 ) ;
#11743=ORIENTED_EDGE ( 'NONE', *, *, #7890, .T. ) ;
#11750=TOROIDAL_SURFACE ( 'NONE', #3681, 40.40389983439752086, 5.000000000000000000 ) ;
#11756=DIRECTION ( 'NONE',  ( 0.000000000000000000, 0.000000000000000000, 1.000000000000000000 ) ) ;
#11757=ORIENTED_EDGE ( 'NONE', *, *, #1942, .F. ) ;
#11773=CARTESIAN_POINT ( 'NONE',  ( -42.53669312409158465, -96.08423613455721579, 5.654315315325685987 ) ) ;
#11798=DIRECTION ( 'NONE',  ( -1.047634945911800068E-14, 0.000000000000000000, 1.000000000000000000 ) ) ;
#11805=DIRECTION ( 'NONE',  ( 0.000000000000000000, 0.000000000000000000, 1.000000000000000000 ) ) ;
#11836=VERTEX_POINT ( 'NONE', #17260 ) ;
#11865=ADVANCED_FACE ( 'NONE', ( #4709 ), #166, .F. ) ;
#11870=ORIENTED_EDGE ( 'NONE', *, *, #7863, .F. ) ;
#11883=ORIENTED_EDGE ( 'NONE', *, *, #233, .F. ) ;
#11885=EDGE_CURVE ( 'NONE', #17089, #9931, #11203, .T. ) ;
#11934=EDGE_LOOP ( 'NONE', ( #11441, #14971, #16345, #10039, #11274 ) ) ;
#11948=DIRECTION ( 'NONE',  ( -0.000000000000000000, -1.000000000000000000, 0.000000000000000000 ) ) ;
#11969=CARTESIAN_POINT ( 'NONE',  ( -115.7702289486888247, -91.08423613455721579, 5.654315315325360913 ) ) ;
#11970=VECTOR ( 'NONE', #9313, 1000.000000000000000 ) ;
#11977=CARTESIAN_POINT ( 'NONE',  ( -60.06546592763100989, -91.08423613455721579, -28.18308811886527110 ) ) ;
#11997=CARTESIAN_POINT ( 'NONE',  ( -115.7073899772186110, -95.23217669033337529, 5.709860480174842046 ) ) ;
#12005=ORIENTED_EDGE ( 'NONE', *, *, #14757, .F. ) ;
#12011=VECTOR ( 'NONE', #1128, 1000.000000000000000 ) ;
#12012=DIRECTION ( 'NONE',  ( 0.000000000000000000, 1.000000000000000000, -0.000000000000000000 ) ) ;
#12022=EDGE_CURVE ( 'NONE', #2924, #16406, #9211, .T. ) ;
#12031=CARTESIAN_POINT ( 'NONE',  ( -76.63889361118792465, -94.42547395655692810, -44.74949031872083083 ) ) ;
#12047=EDGE_LOOP ( 'NONE', ( #11870, #16190, #4618, #8006 ) ) ;
#12069=CARTESIAN_POINT ( 'NONE',  ( -65.06546592763127990, -96.08423613455721579, -2.621725226070001387E-13 ) ) ;
#12071=DIRECTION ( 'NONE',  ( -1.000000000000000000, 0.000000000000000000, -4.029365176583847629E-15 ) ) ;
#12083=CARTESIAN_POINT ( 'NONE',  ( -25.66933353722516031, -95.65021616327642562, -5.654315315325675328 ) ) ;
#12137=EDGE_CURVE ( 'NONE', #13598, #11067, #12421, .T. ) ;
#12143=CARTESIAN_POINT ( 'NONE',  ( -81.37409655828275845, -91.08423613455721579, 28.18308811886534571 ) ) ;
#12147=EDGE_CURVE ( 'NONE', #12706, #15989, #2666, .T. ) ;
#12154=ORIENTED_EDGE ( 'NONE', *, *, #11245, .F. ) ;
#12170=CARTESIAN_POINT ( 'NONE',  ( -70.71978124295668522, -91.08423613455721579, -17.52877280353970235 ) ) ;
#12203=( LENGTH_UNIT ( ) NAMED_UNIT ( * ) SI_UNIT ( .MILLI., .METRE. ) );
#12212=CARTESIAN_POINT ( 'NONE',  ( -77.34864400865002665, -93.09900722835551790, -43.93281456327065371 ) ) ;
#12223=ORIENTED_EDGE ( 'NONE', *, *, #9034, .F. ) ;
#12251=ADVANCED_FACE ( 'NONE', ( #10471 ), #1774, .T. ) ;
#12320=ORIENTED_EDGE ( 'NONE', *, *, #13958, .T. ) ;
#12322=DIRECTION ( 'NONE',  ( -0.000000000000000000, -1.000000000000000000, -0.000000000000000000 ) ) ;
#12378=CARTESIAN_POINT ( 'NONE',  ( -70.71978124295696944, -111.0842361345572158, 5.204170427930421283E-15 ) ) ;
#12389=CARTESIAN_POINT ( 'NONE',  ( -110.0337185876618520, -91.08930958056578220, 10.39386245929412134 ) ) ;
#12407=VECTOR ( 'NONE', #10664, 1000.000000000000000 ) ;
#12421=CIRCLE ( 'NONE', #11517, 5.000000000000004441 ) ;
#12438=AXIS2_PLACEMENT_3D ( 'NONE', #10408, #2691, #11630 ) ;
#12443=CARTESIAN_POINT ( 'NONE',  ( -63.64920489524579494, -92.58099833983884253, 43.41642524957604365 ) ) ;
#12462=CARTESIAN_POINT ( 'NONE',  ( -25.66933353722515676, -96.08423613455721579, -5.654315315325675328 ) ) ;
#12470=DIRECTION ( 'NONE',  ( 0.000000000000000000, 0.000000000000000000, -1.000000000000000000 ) ) ;
#12478=DIRECTION ( 'NONE',  ( 0.000000000000000000, 0.000000000000000000, -1.000000000000000000 ) ) ;
#12481=ORIENTED_EDGE ( 'NONE', *, *, #8337, .T. ) ;
#12490=ADVANCED_FACE ( 'NONE', ( #5604 ), #11326, .T. ) ;
#12497=CARTESIAN_POINT ( 'NONE',  ( -29.41692657362415275, -91.42293623445492301, 8.824457138344833140 ) ) ;
#12502=LINE ( 'NONE', #11086, #4223 ) ;
#12534=ORIENTED_EDGE ( 'NONE', *, *, #939, .T. ) ;
#12545=CARTESIAN_POINT ( 'NONE',  ( -42.53669312409158465, -91.08423613455721579, 10.65431531532568599 ) ) ;
#12571=DIRECTION ( 'NONE',  ( 0.000000000000000000, 1.000000000000000000, -0.000000000000000000 ) ) ;
#12643=AXIS2_PLACEMENT_3D ( 'NONE', #6224, #11948, #10551 ) ;
#12646=CARTESIAN_POINT ( 'NONE',  ( -62.67046908522777926, -91.80659809767261947, -42.25010775664318174 ) ) ;
#12653=CIRCLE ( 'NONE', #12940, 5.000000000000000888 ) ;
#12692=ORIENTED_EDGE ( 'NONE', *, *, #5939, .T. ) ;
#12706=VERTEX_POINT ( 'NONE', #14661 ) ;
#12748=CARTESIAN_POINT ( 'NONE',  ( -61.37143594624207310, -91.24992749556382421, -40.65007029793605398 ) ) ;
#12815=FACE_OUTER_BOUND ( 'NONE', #15296, .T. ) ;
#12817=CARTESIAN_POINT ( 'NONE',  ( -64.65314733921357515, -94.06000665574431707, -44.58117175117413211 ) ) ;
#12821=DIRECTION ( 'NONE',  ( -0.000000000000000000, -1.000000000000000000, -0.000000000000000000 ) ) ;
#12828=VERTEX_POINT ( 'NONE', #2502 ) ;
#12837=UNCERTAINTY_MEASURE_WITH_UNIT (LENGTH_MEASURE( 1.000000000000000082E-05 ), #6501, 'distance_accuracy_value', 'NONE');
#12855=CARTESIAN_POINT ( 'NONE',  ( -113.8539578924277293, -92.35432678654407823, -7.309977258218748553 ) ) ;
#12867=CARTESIAN_POINT ( 'NONE',  ( -81.37409655828275845, -96.08423613455721579, 28.18308811886534571 ) ) ;
#12879=DIRECTION ( 'NONE',  ( -1.040834085586083310E-14, 0.000000000000000000, 1.000000000000000000 ) ) ;
#12882=VECTOR ( 'NONE', #11408, 1000.000000000000000 ) ;
#12940=AXIS2_PLACEMENT_3D ( 'NONE', #1087, #9675, #1166 ) ;
#12944=DIRECTION ( 'NONE',  ( 1.000000000000000000, 0.000000000000000000, 6.950654929607132427E-15 ) ) ;
#12946=CARTESIAN_POINT ( 'NONE',  ( -76.78641432137915501, -94.06000857856479058, 44.58117269483245337 ) ) ;
#12962=CARTESIAN_POINT ( 'NONE',  ( -42.53669312409158465, -91.08423613455721579, 5.654315315325685987 ) ) ;
#12966=CARTESIAN_POINT ( 'NONE',  ( -25.97029152202262026, -94.42547236494613117, 5.919112892686011484 ) ) ;
#13008=CARTESIAN_POINT ( 'NONE',  ( -64.09091675475967520, -93.09900487505510114, -43.93281256380662114 ) ) ;
#13028=CARTESIAN_POINT ( 'NONE',  ( -65.06546592763139358, -96.08423613455721579, 28.18308811886540610 ) ) ;
#13037=CARTESIAN_POINT ( 'NONE',  ( -81.11364370225147979, -91.08930958056578220, 39.31393734470474755 ) ) ;
#13043=CARTESIAN_POINT ( 'NONE',  ( -115.7702289486887395, -96.08423613455721579, -5.654315315326000402 ) ) ;
#13055=SHAPE_REPRESENTATION ( 'Lower Replaceable Die Bushing', ( #16217 ), #17131 ) ;
#13064=ORIENTED_EDGE ( 'NONE', *, *, #3420, .T. ) ;
#13090=LINE ( 'NONE', #5951, #5169 ) ;
#13138=EDGE_CURVE ( 'NONE', #7404, #7872, #5517, .T. ) ;
#13150=DIRECTION ( 'NONE',  ( -3.223492141267075737E-15, 0.000000000000000000, 1.000000000000000000 ) ) ;
#13168=CIRCLE ( 'NONE', #13765, 45.40389983439752086 ) ;
#13189=CARTESIAN_POINT ( 'NONE',  ( -76.37409655828219002, -91.08423613455721579, -45.05044770573186952 ) ) ;
#13191=ORIENTED_EDGE ( 'NONE', *, *, #7918, .T. ) ;
#13192=VECTOR ( 'NONE', #12944, 1000.000000000000000 ) ;
#13200=CYLINDRICAL_SURFACE ( 'NONE', #14636, 5.000000000000004441 ) ;
#13201=DIRECTION ( 'NONE',  ( 4.029365176583844474E-15, -0.000000000000000000, -1.000000000000000000 ) ) ;
#13225=DIRECTION ( 'NONE',  ( -0.000000000000000000, -1.000000000000000000, -0.000000000000000000 ) ) ;
#13237=EDGE_LOOP ( 'NONE', ( #4532, #11721, #8801, #1244, #9218, #14850, #2559, #13283, #6198, #10503, #2949, #13064, #12481, #15298, #2235, #14187, #13191 ) ) ;
#13275=VECTOR ( 'NONE', #17236, 1000.000000000000000 ) ;
#13283=ORIENTED_EDGE ( 'NONE', *, *, #4659, .T. ) ;
#13308=AXIS2_PLACEMENT_3D ( 'NONE', #13635, #6417, #17827 ) ;
#13331=CARTESIAN_POINT ( 'NONE',  ( -25.66933353722515676, -96.08423613455721579, 5.654315315325685987 ) ) ;
#13334=CARTESIAN_POINT ( 'NONE',  ( -42.53669312409158465, -96.08423613455721579, 10.65431531532568599 ) ) ;
#13335=ORIENTED_EDGE ( 'NONE', *, *, #2430, .T. ) ;
#13337=VERTEX_POINT ( 'NONE', #1015 ) ;
#13364=ORIENTED_EDGE ( 'NONE', *, *, #3164, .T. ) ;
#13387=EDGE_CURVE ( 'NONE', #7647, #15598, #16812, .T. ) ;
#13403=CARTESIAN_POINT ( 'NONE',  ( 7.405446926805384449E-14, -96.08423613455721579, -10.65431531532519571 ) ) ;
#13421=ORIENTED_EDGE ( 'NONE', *, *, #2984, .T. ) ;
#13428=CARTESIAN_POINT ( 'NONE',  ( -80.85270481228980088, -91.10977358899566525, -39.65137850708998002 ) ) ;
#13540=CIRCLE ( 'NONE', #18339, 45.40389983439752086 ) ;
#13542=LINE ( 'NONE', #12143, #10280 ) ;
#13550=CARTESIAN_POINT ( 'NONE',  ( -65.06546592763129411, -91.08423613455721579, -6.816485587782003001E-13 ) ) ;
#13560=LINE ( 'NONE', #7748, #12407 ) ;
#13570=CARTESIAN_POINT ( 'NONE',  ( -98.90286936182243949, -96.08423613455721579, 10.65431531532547815 ) ) ;
#13579=AXIS2_PLACEMENT_3D ( 'NONE', #16849, #5430, #9836 ) ;
#13594=CYLINDRICAL_SURFACE ( 'NONE', #17962, 4.999999999999997335 ) ;
#13598=VERTEX_POINT ( 'NONE', #8673 ) ;
#13608=TOROIDAL_SURFACE ( 'NONE', #9133, 10.65431531532568243, 5.000000000000000000 ) ;
#13609=EDGE_CURVE ( 'NONE', #16233, #5685, #11515, .T. ) ;
#13635=CARTESIAN_POINT ( 'NONE',  ( -70.71978124295708312, -96.08423613455721579, 28.18308811886538479 ) ) ;
#13647=CARTESIAN_POINT ( 'NONE',  ( -70.71978124295668522, -91.08423613455721579, -28.18308811886538479 ) ) ;
#13658=LINE ( 'NONE', #10843, #6992 ) ;
#13669=DIRECTION ( 'NONE',  ( 0.000000000000000000, 0.000000000000000000, 1.000000000000000000 ) ) ;
#13684=CARTESIAN_POINT ( 'NONE',  ( -109.8630080638467064, -91.08423613455721579, 10.52500441287563326 ) ) ;
#13687=ORIENTED_EDGE ( 'NONE', *, *, #5146, .F. ) ;
#13692=TOROIDAL_SURFACE ( 'NONE', #5634, 10.65431531532567888, 5.000000000000000000 ) ;
#13700=DIRECTION ( 'NONE',  ( 0.000000000000000000, 0.000000000000000000, 1.000000000000000000 ) ) ;
#13709=EDGE_LOOP ( 'NONE', ( #5535, #16043, #275, #17939 ) ) ;
#13721=AXIS2_PLACEMENT_3D ( 'NONE', #336, #6028, #11756 ) ;
#13730=CARTESIAN_POINT ( 'NONE',  ( -60.06546592763143622, -91.08423613455721579, 38.97384619189705290 ) ) ;
#13758=CARTESIAN_POINT ( 'NONE',  ( -26.78696867915027724, -93.09900487505512956, -6.628864488196836824 ) ) ;
#13765=AXIS2_PLACEMENT_3D ( 'NONE', #15209, #4183, #1297 ) ;
#13784=CARTESIAN_POINT ( 'NONE',  ( -3.930119462002491844E-14, -111.0842361345572158, 5.654315315326165603 ) ) ;
#13792=VECTOR ( 'NONE', #3267, 1000.000000000000000 ) ;
#13827=CARTESIAN_POINT ( 'NONE',  ( -60.32591256472624508, -91.08930925317537231, 39.31392926885263250 ) ) ;
#13868=DIRECTION ( 'NONE',  ( -0.000000000000000000, -1.000000000000000000, -0.000000000000000000 ) ) ;
#13885=CARTESIAN_POINT ( 'NONE',  ( 0.000000000000000000, -96.08423613455721579, 10.65431531532568599 ) ) ;
#13917=LINE ( 'NONE', #9505, #1781 ) ;
#13918=DIRECTION ( 'NONE',  ( 1.000000000000000000, 0.000000000000000000, 0.000000000000000000 ) ) ;
#13920=CARTESIAN_POINT ( 'NONE',  ( -98.90286936182231159, -96.08423613455721579, -5.654315315325883162 ) ) ;
#13921=ORIENTED_EDGE ( 'NONE', *, *, #9320, .F. ) ;
#13948=CARTESIAN_POINT ( 'NONE',  ( -98.90286936182235422, -91.08423613455721579, -2.027180301682503564E-13 ) ) ;
#13953=VERTEX_POINT ( 'NONE', #660 ) ;
#13958=EDGE_CURVE ( 'NONE', #17713, #15472, #10612, .T. ) ;
#13974=ORIENTED_EDGE ( 'NONE', *, *, #10577, .T. ) ;
#13981=EDGE_CURVE ( 'NONE', #3710, #1115, #14783, .T. ) ;
#13982=VERTEX_POINT ( 'NONE', #11977 ) ;
#14027=EDGE_CURVE ( 'NONE', #15074, #14163, #867, .T. ) ;
#14058=VERTEX_POINT ( 'NONE', #15350 ) ;
#14095=ORIENTED_EDGE ( 'NONE', *, *, #9721, .F. ) ;
#14116=CIRCLE ( 'NONE', #10213, 5.654315315325682434 ) ;
#14129=DIRECTION ( 'NONE',  ( 1.000000000000000000, 0.000000000000000000, -0.000000000000000000 ) ) ;
#14130=CARTESIAN_POINT ( 'NONE',  ( -65.06546592763082515, -96.08423613455721579, -45.05044770573174873 ) ) ;
#14149=DIRECTION ( 'NONE',  ( -0.000000000000000000, -1.000000000000000000, 0.000000000000000000 ) ) ;
#14163=VERTEX_POINT ( 'NONE', #5530 ) ;
#14169=CARTESIAN_POINT ( 'NONE',  ( -65.06546592763099568, -96.08423613455721579, -28.18308811886532084 ) ) ;
#14187=ORIENTED_EDGE ( 'NONE', *, *, #14634, .T. ) ;
#14234=CYLINDRICAL_SURFACE ( 'NONE', #4638, 45.40389983439752086 ) ;
#14244=EDGE_LOOP ( 'NONE', ( #15886, #8146, #17973, #2772 ) ) ;
#14267=EDGE_CURVE ( 'NONE', #14163, #6267, #8799, .T. ) ;
#14324=AXIS2_PLACEMENT_3D ( 'NONE', #17129, #14149, #8811 ) ;
#14337=CARTESIAN_POINT ( 'NONE',  ( -77.34864400865063772, -93.09900722835554632, 43.93281456327058265 ) ) ;
#14355=DIRECTION ( 'NONE',  ( 0.000000000000000000, 1.000000000000000000, -0.000000000000000000 ) ) ;
#14360=ORIENTED_EDGE ( 'NONE', *, *, #11885, .F. ) ;
#14383=CARTESIAN_POINT ( 'NONE',  ( -25.66933353722515676, -111.0842361345572158, -5.654315315325675328 ) ) ;
#14384=ORIENTED_EDGE ( 'NONE', *, *, #9031, .F. ) ;
#14393=CARTESIAN_POINT ( 'NONE',  ( -61.89532410461173129, -91.42293623445490880, -41.30285466933271010 ) ) ;
#14403=CARTESIAN_POINT ( 'NONE',  ( -42.53669312409158465, -91.08423613455721579, 10.65431531532568599 ) ) ;
#14458=ORIENTED_EDGE ( 'NONE', *, *, #16595, .F. ) ;
#14459=EDGE_LOOP ( 'NONE', ( #7080, #153, #8621, #4941 ) ) ;
#14469=DIRECTION ( 'NONE',  ( 0.000000000000000000, 0.000000000000000000, 1.000000000000000000 ) ) ;
#14478=DIRECTION ( 'NONE',  ( -0.000000000000000000, -1.000000000000000000, 0.000000000000000000 ) ) ;
#14489=ORIENTED_EDGE ( 'NONE', *, *, #1307, .T. ) ;
#14593=LINE ( 'NONE', #8547, #9920 ) ;
#14613=DIRECTION ( 'NONE',  ( 0.000000000000000000, 1.000000000000000000, -0.000000000000000000 ) ) ;
#14634=EDGE_CURVE ( 'NONE', #17089, #11153, #18222, .T. ) ;
#14636=AXIS2_PLACEMENT_3D ( 'NONE', #380, #11798, #17486 ) ;
#14641=ORIENTED_EDGE ( 'NONE', *, *, #6143, .T. ) ;
#14661=CARTESIAN_POINT ( 'NONE',  ( -65.06546592763146464, -96.08423613455721579, 45.05044770573184110 ) ) ;
#14688=CARTESIAN_POINT ( 'NONE',  ( -70.71978124295708312, -111.0842361345572158, 28.18308811886538479 ) ) ;
#14717=ORIENTED_EDGE ( 'NONE', *, *, #7000, .T. ) ;
#14728=EDGE_LOOP ( 'NONE', ( #9793, #2931, #9926, #15938 ) ) ;
#14737=ADVANCED_FACE ( 'NONE', ( #3159 ), #1740, .F. ) ;
#14757=EDGE_CURVE ( 'NONE', #15598, #14963, #6491, .T. ) ;
#14783=CIRCLE ( 'NONE', #16890, 40.40389983439752086 ) ;
#14790=EDGE_CURVE ( 'NONE', #13337, #7261, #3912, .T. ) ;
#14802=DIRECTION ( 'NONE',  ( -0.000000000000000000, -1.000000000000000000, -0.000000000000000000 ) ) ;
#14803=ORIENTED_EDGE ( 'NONE', *, *, #11245, .T. ) ;
#14812=EDGE_CURVE ( 'NONE', #5095, #3710, #8975, .T. ) ;
#14817=ORIENTED_EDGE ( 'NONE', *, *, #6991, .F. ) ;
#14829=FACE_OUTER_BOUND ( 'NONE', #6833, .T. ) ;
#14841=DIRECTION ( 'NONE',  ( 4.029365176583844474E-15, 0.000000000000000000, -1.000000000000000000 ) ) ;
#14850=ORIENTED_EDGE ( 'NONE', *, *, #13981, .T. ) ;
#14890=CARTESIAN_POINT ( 'NONE',  ( -114.8884567811963677, -93.39009998357855125, 6.425136209963392631 ) ) ;
#14899=DIRECTION ( 'NONE',  ( -1.000000000000000000, 0.000000000000000000, -1.110223024625157172E-14 ) ) ;
#14900=DIRECTION ( 'NONE',  ( 1.047634945911799279E-14, -0.000000000000000000, -1.000000000000000000 ) ) ;
#14902=DIRECTION ( 'NONE',  ( -1.000000000000000000, 0.000000000000000000, 0.000000000000000000 ) ) ;
#14906=DIRECTION ( 'NONE',  ( -1.000000000000000000, 0.000000000000000000, 0.000000000000000000 ) ) ;
#14918=( NAMED_UNIT ( * ) SI_UNIT ( $, .STERADIAN. ) SOLID_ANGLE_UNIT ( ) );
#14922=LINE ( 'NONE', #17642, #17931 ) ;
#14937=LINE ( 'NONE', #10661, #9359 ) ;
#14940=PLANE ( 'NONE',  #3725 ) ;
#14953=ORIENTED_EDGE ( 'NONE', *, *, #9596, .T. ) ;
#14957=CARTESIAN_POINT ( 'NONE',  ( -31.74593505105995916, -91.08423613455721579, -10.65431531532567710 ) ) ;
#14960=EDGE_CURVE ( 'NONE', #5095, #7404, #13917, .T. ) ;
#14963=VERTEX_POINT ( 'NONE', #3989 ) ;
#14971=ORIENTED_EDGE ( 'NONE', *, *, #16960, .F. ) ;
#14978=FACE_OUTER_BOUND ( 'NONE', #17044, .T. ) ;
#14989=AXIS2_PLACEMENT_3D ( 'NONE', #696, #7624, #7979 ) ;
#15000=AXIS2_PLACEMENT_3D ( 'NONE', #875, #17611, #17804 ) ;
#15004=DIRECTION ( 'NONE',  ( 0.000000000000000000, -0.000000000000000000, 1.000000000000000000 ) ) ;
#15006=CIRCLE ( 'NONE', #11160, 40.40389983439752086 ) ;
#15009=CARTESIAN_POINT ( 'NONE',  ( -70.71978124295696944, -91.08423613455721579, 5.204170427930421283E-15 ) ) ;
#15012=VECTOR ( 'NONE', #6216, 1000.000000000000000 ) ;
#15017=AXIS2_PLACEMENT_3D ( 'NONE', #18147, #1214, #14129 ) ;
#15052=LINE ( 'NONE', #11969, #13792 ) ;
#15059=CARTESIAN_POINT ( 'NONE',  ( -28.46967348631369177, -91.80659809767261947, -8.049312157728762074 ) ) ;
#15065=ORIENTED_EDGE ( 'NONE', *, *, #11587, .F. ) ;
#15066=PRODUCT_DEFINITION_CONTEXT ( 'detailed design', #7176, 'design' ) ;
#15067=CARTESIAN_POINT ( 'NONE',  ( -98.90286936182239685, -96.08423613455721579, 5.654315315325477265 ) ) ;
#15074=VERTEX_POINT ( 'NONE', #5855 ) ;
#15077=DIRECTION ( 'NONE',  ( 0.000000000000000000, 1.000000000000000000, -0.000000000000000000 ) ) ;
#15080=AXIS2_PLACEMENT_3D ( 'NONE', #11246, #16931, #17286 ) ;
#15108=EDGE_CURVE ( 'NONE', #5840, #3816, #16290, .T. ) ;
#15110=DIRECTION ( 'NONE',  ( 0.000000000000000000, 0.000000000000000000, 1.000000000000000000 ) ) ;
#15136=EDGE_LOOP ( 'NONE', ( #9972, #11113, #13335, #11361 ) ) ;
#15166=DIRECTION ( 'NONE',  ( 0.000000000000000000, 0.000000000000000000, -1.000000000000000000 ) ) ;
#15173=ORIENTED_EDGE ( 'NONE', *, *, #17259, .F. ) ;
#15178=ORIENTED_EDGE ( 'NONE', *, *, #14267, .F. ) ;
#15202=DIRECTION ( 'NONE',  ( -1.047634945911800068E-14, 0.000000000000000000, 1.000000000000000000 ) ) ;
#15209=CARTESIAN_POINT ( 'NONE',  ( -70.71978124295696944, -96.08423613455721579, 5.204170427930421283E-15 ) ) ;
#15219=CARTESIAN_POINT ( 'NONE',  ( -60.58685171690505200, -91.10977296152353233, 39.65137083761684522 ) ) ;
#15240=ADVANCED_FACE ( 'NONE', ( #9552 ), #2075, .F. ) ;
#15271=AXIS2_PLACEMENT_3D ( 'NONE', #10902, #701, #2276 ) ;
#15272=LINE ( 'NONE', #13784, #3824 ) ;
#15282=CARTESIAN_POINT ( 'NONE',  ( -31.57667891805219895, -91.08423613455724421, 10.52509945732312957 ) ) ;
#15290=CARTESIAN_POINT ( 'NONE',  ( -76.37409655828275845, -91.08423613455721579, 28.18308811886536347 ) ) ;
#15292=AXIS2_PLACEMENT_3D ( 'NONE', #4286, #15958, #9996 ) ;
#15296=EDGE_LOOP ( 'NONE', ( #15178, #16018, #10985, #16361 ) ) ;
#15298=ORIENTED_EDGE ( 'NONE', *, *, #14790, .T. ) ;
#15299=DIRECTION ( 'NONE',  ( 0.000000000000000000, 0.000000000000000000, 1.000000000000000000 ) ) ;
#15316=CARTESIAN_POINT ( 'NONE',  ( -62.92154743286889129, -91.96845925178436687, 42.55229934223208943 ) ) ;
#15329=ORIENTED_EDGE ( 'NONE', *, *, #10663, .F. ) ;
#15331=PLANE ( 'NONE',  #15017 ) ;
#15347=DIRECTION ( 'NONE',  ( 8.326672684688674053E-15, 0.000000000000000000, -1.000000000000000000 ) ) ;
#15350=CARTESIAN_POINT ( 'NONE',  ( -98.90286936182239685, -111.0842361345572158, 5.654315315325477265 ) ) ;
#15361=CARTESIAN_POINT ( 'NONE',  ( -70.71978124295696944, -91.08423613455721579, 5.204170427930421283E-15 ) ) ;
#15391=CARTESIAN_POINT ( 'NONE',  ( -65.06546592763146464, -91.08423613455721579, 45.05044770573184110 ) ) ;
#15451=EDGE_LOOP ( 'NONE', ( #5838, #7952, #17223, #3499 ) ) ;
#15467=CARTESIAN_POINT ( 'NONE',  ( -70.71978124295696944, -111.0842361345572158, 5.204170427930421283E-15 ) ) ;
#15472=VERTEX_POINT ( 'NONE', #8813 ) ;
#15496=DIRECTION ( 'NONE',  ( 0.000000000000000000, 0.000000000000000000, -1.000000000000000000 ) ) ;
#15546=DIRECTION ( 'NONE',  ( -1.000000000000000000, 2.888894916580850627E-30, -8.326672684688672475E-15 ) ) ;
#15563=ADVANCED_FACE ( 'NONE', ( #7482 ), #13200, .T. ) ;
#15566=DIRECTION ( 'NONE',  ( 0.000000000000000000, 0.000000000000000000, -1.000000000000000000 ) ) ;
#15583=DIRECTION ( 'NONE',  ( 0.000000000000000000, 0.000000000000000000, 1.000000000000000000 ) ) ;
#15596=EDGE_CURVE ( 'NONE', #12706, #800, #7752, .T. ) ;
#15598=VERTEX_POINT ( 'NONE', #10569 ) ;
#15624=CARTESIAN_POINT ( 'NONE',  ( -63.64920489524519809, -92.58099833983887095, -43.41642524957592997 ) ) ;
#15688=AXIS2_PLACEMENT_3D ( 'NONE', #7714, #18008, #9134 ) ;
#15707=ORIENTED_EDGE ( 'NONE', *, *, #17726, .F. ) ;
#15729=EDGE_LOOP ( 'NONE', ( #12223, #2370, #13421, #17560 ) ) ;
#15736=EDGE_LOOP ( 'NONE', ( #3018, #6588, #3607, #3535 ) ) ;
#15747=EDGE_LOOP ( 'NONE', ( #15811, #8744, #7117, #17576 ) ) ;
#15771=ORIENTED_EDGE ( 'NONE', *, *, #9396, .F. ) ;
#15811=ORIENTED_EDGE ( 'NONE', *, *, #14812, .T. ) ;
#15825=CARTESIAN_POINT ( 'NONE',  ( -78.02975850117555012, -92.35432678654406402, 43.13417664947079544 ) ) ;
#15828=EDGE_LOOP ( 'NONE', ( #1822, #7068, #6324, #5865 ) ) ;
#15845=CARTESIAN_POINT ( 'NONE',  ( -70.71978124295708312, -96.08423613455721579, 22.52877280353970235 ) ) ;
#15870=AXIS2_PLACEMENT_3D ( 'NONE', #16395, #14902, #705 ) ;
#15886=ORIENTED_EDGE ( 'NONE', *, *, #6210, .F. ) ;
#15899=VECTOR ( 'NONE', #18242, 1000.000000000000000 ) ;
#15938=ORIENTED_EDGE ( 'NONE', *, *, #5939, .F. ) ;
#15958=DIRECTION ( 'NONE',  ( -0.000000000000000000, -1.000000000000000000, 0.000000000000000000 ) ) ;
#15989=VERTEX_POINT ( 'NONE', #6606 ) ;
#16007=EDGE_CURVE ( 'NONE', #7696, #13982, #14922, .T. ) ;
#16018=ORIENTED_EDGE ( 'NONE', *, *, #4027, .T. ) ;
#16025=CARTESIAN_POINT ( 'NONE',  ( -70.71978124295696944, -91.08423613455721579, 5.204170427930421283E-15 ) ) ;
#16043=ORIENTED_EDGE ( 'NONE', *, *, #12022, .F. ) ;
#16115=EDGE_CURVE ( 'NONE', #16406, #14163, #13168, .T. ) ;
#16143=VECTOR ( 'NONE', #13225, 1000.000000000000000 ) ;
#16190=ORIENTED_EDGE ( 'NONE', *, *, #8108, .F. ) ;
#16192=DIRECTION ( 'NONE',  ( -1.000000000000000000, 0.000000000000000000, -1.047634945911799121E-14 ) ) ;
#16217=AXIS2_PLACEMENT_3D ( 'NONE', #5781, #6037, #8961 ) ;
#16233=VERTEX_POINT ( 'NONE', #11651 ) ;
#16250=VERTEX_POINT ( 'NONE', #4282 ) ;
#16263=VECTOR ( 'NONE', #5177, 1000.000000000000000 ) ;
#16267=AXIS2_PLACEMENT_3D ( 'NONE', #6071, #13201, #12071 ) ;
#16290=LINE ( 'NONE', #17085, #11058 ) ;
#16295=CARTESIAN_POINT ( 'NONE',  ( -7.405446926806058452E-14, -96.08423613455721579, 10.65431531532616560 ) ) ;
#16298=CYLINDRICAL_SURFACE ( 'NONE', #8755, 5.000000000000000000 ) ;
#16338=CARTESIAN_POINT ( 'NONE',  ( -64.65314733921417201, -94.06000665574430286, 44.58117175117424580 ) ) ;
#16345=ORIENTED_EDGE ( 'NONE', *, *, #1307, .F. ) ;
#16361=ORIENTED_EDGE ( 'NONE', *, *, #17608, .F. ) ;
#16373=ORIENTED_EDGE ( 'NONE', *, *, #7425, .F. ) ;
#16376=EDGE_LOOP ( 'NONE', ( #16391, #4846, #9009, #5328 ) ) ;
#16391=ORIENTED_EDGE ( 'NONE', *, *, #5621, .T. ) ;
#16395=CARTESIAN_POINT ( 'NONE',  ( 0.000000000000000000, -96.08423613455721579, -10.65431531532567710 ) ) ;
#16398=VECTOR ( 'NONE', #48, 1000.000000000000000 ) ;
#16400=PLANE ( 'NONE',  #17687 ) ;
#16406=VERTEX_POINT ( 'NONE', #6296 ) ;
#16411=ORIENTED_EDGE ( 'NONE', *, *, #10528, .F. ) ;
#16424=B_SPLINE_CURVE_WITH_KNOTS ( 'NONE', 3,
 ( #966, #6667, #11997, #4974, #3384, #14890, #10781, #1992, #3570, #7970, #3485, #5164, #16476, #9109, #7881, #10688, #10879, #12389, #13684, #10604 ),
 .UNSPECIFIED., .F., .F.,
 ( 4, 2, 2, 2, 2, 2, 2, 2, 2, 4 ),
 ( 0.000000000000000000, 0.001278592738658798026, 0.002557185477317596052, 0.003835778215976394078, 0.005114370954635192104, 0.006392963693293989696, 0.007671556431952788156, 0.008950149170611586616, 0.009589445539940984545, 0.01022874190927038421 ),
 .UNSPECIFIED. ) ;
#16434=ADVANCED_FACE ( 'NONE', ( #4711 ), #3311, .T. ) ;
#16454=CARTESIAN_POINT ( 'NONE',  ( -26.55110732739451507, -93.39009773859100960, -6.425137615056142337 ) ) ;
#16459=ADVANCED_FACE ( 'NONE', ( #2006 ), #2280, .T. ) ;
#16466=DIRECTION ( 'NONE',  ( 0.000000000000000000, 0.000000000000000000, 1.000000000000000000 ) ) ;
#16467=EDGE_CURVE ( 'NONE', #16250, #800, #17945, .T. ) ;
#16476=CARTESIAN_POINT ( 'NONE',  ( -112.0226416184558076, -91.42293805878655633, 8.824452519952380669 ) ) ;
#16502=VECTOR ( 'NONE', #14906, 1000.000000000000000 ) ;
#16547=DIRECTION ( 'NONE',  ( 3.223492141267075737E-15, 0.000000000000000000, -1.000000000000000000 ) ) ;
#16572=VERTEX_POINT ( 'NONE', #2763 ) ;
#16576=CARTESIAN_POINT ( 'NONE',  ( -70.71978124295696944, -91.08423613455721579, 5.204170427930421283E-15 ) ) ;
#16595=EDGE_CURVE ( 'NONE', #11655, #17058, #12502, .T. ) ;
#16615=DIRECTION ( 'NONE',  ( -1.047634945911799279E-14, 0.000000000000000000, 1.000000000000000000 ) ) ;
#16637=FACE_OUTER_BOUND ( 'NONE', #1629, .T. ) ;
#16641=CARTESIAN_POINT ( 'NONE',  ( -29.09351669014244379, -91.53392936304807392, -8.561724358915437705 ) ) ;
#16702=DIRECTION ( 'NONE',  ( 0.000000000000000000, 1.000000000000000000, -0.000000000000000000 ) ) ;
#16709=CARTESIAN_POINT ( 'NONE',  ( -64.29464362790101006, -93.39009773859098118, 44.16867391556250766 ) ) ;
#16714=CIRCLE ( 'NONE', #3278, 45.40389983439752086 ) ;
#16718=DIRECTION ( 'NONE',  ( 6.950654929607132427E-15, 0.000000000000000000, -1.000000000000000000 ) ) ;
#16725=AXIS2_PLACEMENT_3D ( 'NONE', #13948, #5420, #759 ) ;
#16726=CARTESIAN_POINT ( 'NONE',  ( -70.71978124295696944, -96.08423613455721579, 5.204170427930421283E-15 ) ) ;
#16729=DIRECTION ( 'NONE',  ( 1.000000000000000000, -0.000000000000000000, 8.326672684688672475E-15 ) ) ;
#16736=AXIS2_PLACEMENT_3D ( 'NONE', #13570, #16729, #15347 ) ;
#16740=DIRECTION ( 'NONE',  ( -3.223492141267075737E-15, -0.000000000000000000, 1.000000000000000000 ) ) ;
#16780=LINE ( 'NONE', #15290, #8448 ) ;
#16783=EDGE_CURVE ( 'NONE', #7936, #17713, #3034, .T. ) ;
#16812=LINE ( 'NONE', #5587, #432 ) ;
#16826=CARTESIAN_POINT ( 'NONE',  ( -109.6936274348538944, -91.08423613455721579, -10.65431531532595777 ) ) ;
#16828=ADVANCED_FACE ( 'NONE', ( #7879 ), #13594, .T. ) ;
#16845=ORIENTED_EDGE ( 'NONE', *, *, #2403, .T. ) ;
#16849=CARTESIAN_POINT ( 'NONE',  ( -70.71978124295708312, -91.08423613455721579, 28.18308811886538479 ) ) ;
#16865=FACE_OUTER_BOUND ( 'NONE', #16376, .T. ) ;
#16890=AXIS2_PLACEMENT_3D ( 'NONE', #17498, #4679, #4759 ) ;
#16925=CARTESIAN_POINT ( 'NONE',  ( -61.10958520376109249, -91.18731141006415442, -40.31989393471889116 ) ) ;
#16931=DIRECTION ( 'NONE',  ( 1.000000000000000000, -0.000000000000000000, 1.047634945911800068E-14 ) ) ;
#16941=ORIENTED_EDGE ( 'NONE', *, *, #10063, .T. ) ;
#16960=EDGE_CURVE ( 'NONE', #4074, #11067, #14116, .T. ) ;
#16982=TOROIDAL_SURFACE ( 'NONE', #8012, 10.65431531532568243, 5.000000000000000000 ) ;
#16992=ORIENTED_EDGE ( 'NONE', *, *, #5621, .F. ) ;
#16995=CARTESIAN_POINT ( 'NONE',  ( -98.90286936182235422, -111.0842361345572158, -2.027180301682503564E-13 ) ) ;
#17020=CIRCLE ( 'NONE', #5667, 5.654315315325682434 ) ;
#17040=LINE ( 'NONE', #2840, #13192 ) ;
#17044=EDGE_LOOP ( 'NONE', ( #14717, #8865, #16992, #9774 ) ) ;
#17049=CARTESIAN_POINT ( 'NONE',  ( -112.0226416184556797, -91.42293805878655633, -8.824452519952979301 ) ) ;
#17058=VERTEX_POINT ( 'NONE', #18171 ) ;
#17068=DIRECTION ( 'NONE',  ( 0.000000000000000000, 1.000000000000000000, -0.000000000000000000 ) ) ;
#17073=CARTESIAN_POINT ( 'NONE',  ( -70.71978124295668522, -96.08423613455721579, -28.18308811886538479 ) ) ;
#17085=CARTESIAN_POINT ( 'NONE',  ( -115.7702289486887395, -91.08423613455721579, -5.654315315326000402 ) ) ;
#17089=VERTEX_POINT ( 'NONE', #14403 ) ;
#17095=VECTOR ( 'NONE', #14841, 1000.000000000000000 ) ;
#17112=FACE_OUTER_BOUND ( 'NONE', #8856, .T. ) ;
#17116=DIRECTION ( 'NONE',  ( 0.000000000000000000, 0.000000000000000000, 1.000000000000000000 ) ) ;
#17129=CARTESIAN_POINT ( 'NONE',  ( -70.71978124295708312, -91.08423613455721579, 28.18308811886538479 ) ) ;
#17131=( GEOMETRIC_REPRESENTATION_CONTEXT ( 3 ) GLOBAL_UNCERTAINTY_ASSIGNED_CONTEXT ( ( #12837 ) ) GLOBAL_UNIT_ASSIGNED_CONTEXT ( ( #6501, #5100, #14918 ) ) REPRESENTATION_CONTEXT ( 'NONE', 'WORKASPACE' ) );
#17135=DIRECTION ( 'NONE',  ( -1.047634945911799279E-14, 0.000000000000000000, 1.000000000000000000 ) ) ;
#17139=CARTESIAN_POINT ( 'NONE',  ( -80.72210053294904242, -91.12516209206944495, 39.81919198398647097 ) ) ;
#17151=DIRECTION ( 'NONE',  ( 1.000000000000000000, -0.000000000000000000, -0.000000000000000000 ) ) ;
#17171=DIRECTION ( 'NONE',  ( 1.000000000000000000, 0.000000000000000000, 1.040834085586083310E-14 ) ) ;
#17190=AXIS2_PLACEMENT_3D ( 'NONE', #14688, #9183, #17577 ) ;
#17205=ORIENTED_EDGE ( 'NONE', *, *, #14790, .F. ) ;
#17216=EDGE_LOOP ( 'NONE', ( #12154, #12692, #1577, #11757 ) ) ;
#17223=ORIENTED_EDGE ( 'NONE', *, *, #4684, .F. ) ;
#17236=DIRECTION ( 'NONE',  ( -0.000000000000000000, -1.000000000000000000, -0.000000000000000000 ) ) ;
#17259=EDGE_CURVE ( 'NONE', #15989, #7936, #9154, .T. ) ;
#17260=CARTESIAN_POINT ( 'NONE',  ( -76.37409655828280108, -96.08423613455721579, 45.05044770573179846 ) ) ;
#17286=DIRECTION ( 'NONE',  ( 1.047634945911800068E-14, 0.000000000000000000, -1.000000000000000000 ) ) ;
#17324=DIRECTION ( 'NONE',  ( 1.000000000000000000, 0.000000000000000000, 3.223492141267071398E-15 ) ) ;
#17329=AXIS2_PLACEMENT_3D ( 'NONE', #13647, #17926, #5218 ) ;
#17359=LINE ( 'NONE', #1571, #4572 ) ;
#17404=DIRECTION ( 'NONE',  ( 0.000000000000000000, 0.000000000000000000, 1.000000000000000000 ) ) ;
#17416=LINE ( 'NONE', #10685, #16143 ) ;
#17426=AXIS2_PLACEMENT_3D ( 'NONE', #3775, #6678, #15566 ) ;
#17456=ORIENTED_EDGE ( 'NONE', *, *, #16783, .T. ) ;
#17476=ORIENTED_EDGE ( 'NONE', *, *, #16783, .F. ) ;
#17486=DIRECTION ( 'NONE',  ( 1.000000000000000000, 0.000000000000000000, 1.047634945911799595E-14 ) ) ;
#17498=CARTESIAN_POINT ( 'NONE',  ( -70.71978124295696944, -91.08423613455721579, 5.204170427930421283E-15 ) ) ;
#17513=FACE_OUTER_BOUND ( 'NONE', #9479, .T. ) ;
#17560=ORIENTED_EDGE ( 'NONE', *, *, #10988, .F. ) ;
#17576=ORIENTED_EDGE ( 'NONE', *, *, #14960, .F. ) ;
#17577=DIRECTION ( 'NONE',  ( 0.000000000000000000, 0.000000000000000000, 1.000000000000000000 ) ) ;
#17592=FACE_OUTER_BOUND ( 'NONE', #787, .T. ) ;
#17608=EDGE_CURVE ( 'NONE', #6267, #7322, #9216, .T. ) ;
#17611=DIRECTION ( 'NONE',  ( 0.000000000000000000, 1.000000000000000000, -0.000000000000000000 ) ) ;
#17617=ADVANCED_FACE ( 'NONE', ( #17813 ), #16400, .F. ) ;
#17629=CIRCLE ( 'NONE', #16725, 10.65431531532567888 ) ;
#17642=CARTESIAN_POINT ( 'NONE',  ( -60.06546592763099568, -91.08423613455721579, -28.18308811886527110 ) ) ;
#17647=ORIENTED_EDGE ( 'NONE', *, *, #17820, .F. ) ;
#17657=AXIS2_PLACEMENT_3D ( 'NONE', #4774, #10875, #12478 ) ;
#17665=DIRECTION ( 'NONE',  ( 4.029365176583844474E-15, 0.000000000000000000, -1.000000000000000000 ) ) ;
#17687=AXIS2_PLACEMENT_3D ( 'NONE', #9309, #15004, #799 ) ;
#17692=DIRECTION ( 'NONE',  ( 6.950654929607131638E-15, 0.000000000000000000, -1.000000000000000000 ) ) ;
#17713=VERTEX_POINT ( 'NONE', #18112 ) ;
#17726=EDGE_CURVE ( 'NONE', #11067, #15472, #16780, .T. ) ;
#17729=CLOSED_SHELL ( 'NONE', ( #1778, #690, #5036, #12490, #1528, #15240, #8823, #1055, #10262, #11865, #10873, #1855, #6817, #17617, #18064, #18445, #2882, #5086, #16434, #14737, #6523, #5670, #7657, #12251, #6756, #10696, #5597, #5498, #10318, #6182, #5478, #16459, #15563, #373, #215, #16828 ) ) ;
#17730=CARTESIAN_POINT ( 'NONE',  ( -77.14491745292022529, -93.39009998357853704, -44.16867553823941961 ) ) ;
#17740=DIRECTION ( 'NONE',  ( 0.000000000000000000, 0.000000000000000000, -1.000000000000000000 ) ) ;
#17757=EDGE_CURVE ( 'NONE', #12828, #5881, #1273, .T. ) ;
#17765=EDGE_LOOP ( 'NONE', ( #7075, #6300, #9297, #9296 ) ) ;
#17779=DIRECTION ( 'NONE',  ( 0.000000000000000000, 0.000000000000000000, 1.000000000000000000 ) ) ;
#17793=DIRECTION ( 'NONE',  ( 1.000000000000000000, 0.000000000000000000, 6.950654929607132427E-15 ) ) ;
#17804=DIRECTION ( 'NONE',  ( 0.000000000000000000, 0.000000000000000000, 1.000000000000000000 ) ) ;
#17813=FACE_OUTER_BOUND ( 'NONE', #7966, .T. ) ;
#17820=EDGE_CURVE ( 'NONE', #15989, #15598, #9641, .T. ) ;
#17827=DIRECTION ( 'NONE',  ( 0.000000000000000000, 0.000000000000000000, 1.000000000000000000 ) ) ;
#17829=DIRECTION ( 'NONE',  ( 3.223492141267075737E-15, -0.000000000000000000, -1.000000000000000000 ) ) ;
#17830=EDGE_LOOP ( 'NONE', ( #13364, #13921, #7877, #6124, #830, #12005, #17647, #18432, #17456, #12320, #15329, #7336, #3140, #6201, #14817, #18518, #12534 ) ) ;
#17849=VERTEX_POINT ( 'NONE', #6261 ) ;
#17864=AXIS2_PLACEMENT_3D ( 'NONE', #1157, #3954, #9667 ) ;
#17895=( NAMED_UNIT ( * ) SI_UNIT ( $, .STERADIAN. ) SOLID_ANGLE_UNIT ( ) );
#17926=DIRECTION ( 'NONE',  ( -0.000000000000000000, -1.000000000000000000, -0.000000000000000000 ) ) ;
#17931=VECTOR ( 'NONE', #16615, 1000.000000000000000 ) ;
#17939=ORIENTED_EDGE ( 'NONE', *, *, #16007, .F. ) ;
#17945=CIRCLE ( 'NONE', #3305, 4.999999999999997335 ) ;
#17957=DIRECTION ( 'NONE',  ( 0.000000000000000000, 1.000000000000000000, -0.000000000000000000 ) ) ;
#17962=AXIS2_PLACEMENT_3D ( 'NONE', #6092, #4775, #16192 ) ;
#17973=ORIENTED_EDGE ( 'NONE', *, *, #6768, .T. ) ;
#17984=DIRECTION ( 'NONE',  ( 1.000000000000000000, 0.000000000000000000, 6.950654929607132427E-15 ) ) ;
#17995=CARTESIAN_POINT ( 'NONE',  ( -60.06546592763100278, -96.08423613455721579, -28.18308811886526755 ) ) ;
#18008=DIRECTION ( 'NONE',  ( 0.000000000000000000, 1.000000000000000000, -0.000000000000000000 ) ) ;
#18032=CARTESIAN_POINT ( 'NONE',  ( -60.19468178563425198, -91.08423613455723000, 39.14310232490466035 ) ) ;
#18058=EDGE_CURVE ( 'NONE', #5881, #9725, #15006, .T. ) ;
#18064=ADVANCED_FACE ( 'NONE', ( #8544 ), #2554, .F. ) ;
#18112=CARTESIAN_POINT ( 'NONE',  ( -70.71978124295708312, -111.0842361345572158, 22.52877280353970235 ) ) ;
#18131=CARTESIAN_POINT ( 'NONE',  ( -31.74593505105995916, -91.08423613455721579, 10.65431531532568599 ) ) ;
#18135=CARTESIAN_POINT ( 'NONE',  ( -64.09091675476031469, -93.09900487505517219, 43.93281256380674193 ) ) ;
#18147=CARTESIAN_POINT ( 'NONE',  ( 0.000000000000000000, -91.08423613455721579, -5.654315315325675328 ) ) ;
#18156=CARTESIAN_POINT ( 'NONE',  ( -25.97029152202262026, -94.42547236494613117, -5.919112892686000826 ) ) ;
#18161=LINE ( 'NONE', #5332, #2813 ) ;
#18171=CARTESIAN_POINT ( 'NONE',  ( -98.90286936182231159, -111.0842361345572158, -5.654315315325883162 ) ) ;
#18185=FACE_OUTER_BOUND ( 'NONE', #17765, .T. ) ;
#18191=CARTESIAN_POINT ( 'NONE',  ( -29.09351669014244379, -91.53392936304807392, 8.561724358915446587 ) ) ;
#18195=DIRECTION ( 'NONE',  ( -0.000000000000000000, -1.000000000000000000, -0.000000000000000000 ) ) ;
#18222=CIRCLE ( 'NONE', #10435, 10.65431531532567888 ) ;
#18242=DIRECTION ( 'NONE',  ( -1.000000000000000000, 0.000000000000000000, 0.000000000000000000 ) ) ;
#18266=CARTESIAN_POINT ( 'NONE',  ( -70.71978124295708312, -96.08423613455721579, 28.18308811886538479 ) ) ;
#18273=AXIS2_PLACEMENT_3D ( 'NONE', #5651, #17068, #4347 ) ;
#18286=ORIENTED_EDGE ( 'NONE', *, *, #12137, .F. ) ;
#18297=DIRECTION ( 'NONE',  ( -1.000000000000000000, -0.000000000000000000, -6.950654929607132427E-15 ) ) ;
#18327=DIRECTION ( 'NONE',  ( -0.000000000000000000, -1.000000000000000000, -0.000000000000000000 ) ) ;
#18339=AXIS2_PLACEMENT_3D ( 'NONE', #11508, #343, #1840 ) ;
#18344=CARTESIAN_POINT ( 'NONE',  ( -62.92154743286826601, -91.96845925178435266, -42.55229934223195443 ) ) ;
#18358=CARTESIAN_POINT ( 'NONE',  ( -115.7702289486887395, -96.08423613455721579, -5.654315315326000402 ) ) ;
#18370=AXIS2_PLACEMENT_3D ( 'NONE', #2185, #12012, #6288 ) ;
#18381=PRODUCT ( 'Lower Replaceable Die Bushing', 'Lower Replaceable Die Bushing', '', ( #9480 ) ) ;
#18392=CARTESIAN_POINT ( 'NONE',  ( -31.74593505105995916, -91.08423613455721579, 10.65431531532568599 ) ) ;
#18432=ORIENTED_EDGE ( 'NONE', *, *, #17259, .T. ) ;
#18435=CARTESIAN_POINT ( 'NONE',  ( -64.29464362790038479, -93.39009773859099539, -44.16867391556240108 ) ) ;
#18445=ADVANCED_FACE ( 'NONE', ( #12815 ), #15331, .T. ) ;
#18508=CARTESIAN_POINT ( 'NONE',  ( -98.90286936182226896, -91.08423613455721579, -10.65431531532588316 ) ) ;
#18518=ORIENTED_EDGE ( 'NONE', *, *, #10577, .F. ) ;
#18539=COLOUR_RGB('Light Blue',0.38,0.62,0.78);
#18540=FILL_AREA_STYLE_COLOUR('',#18539);
#18541=FILL_AREA_STYLE('',(#18540));
#18542=SURFACE_STYLE_FILL_AREA(#18541);
#18543=SURFACE_SIDE_STYLE('',(#18542));
#18544=SURFACE_STYLE_USAGE(.BOTH.,#18543);
#18545=PRESENTATION_STYLE_ASSIGNMENT((#18544));
ENDSEC;
END-ISO-10303-21;
